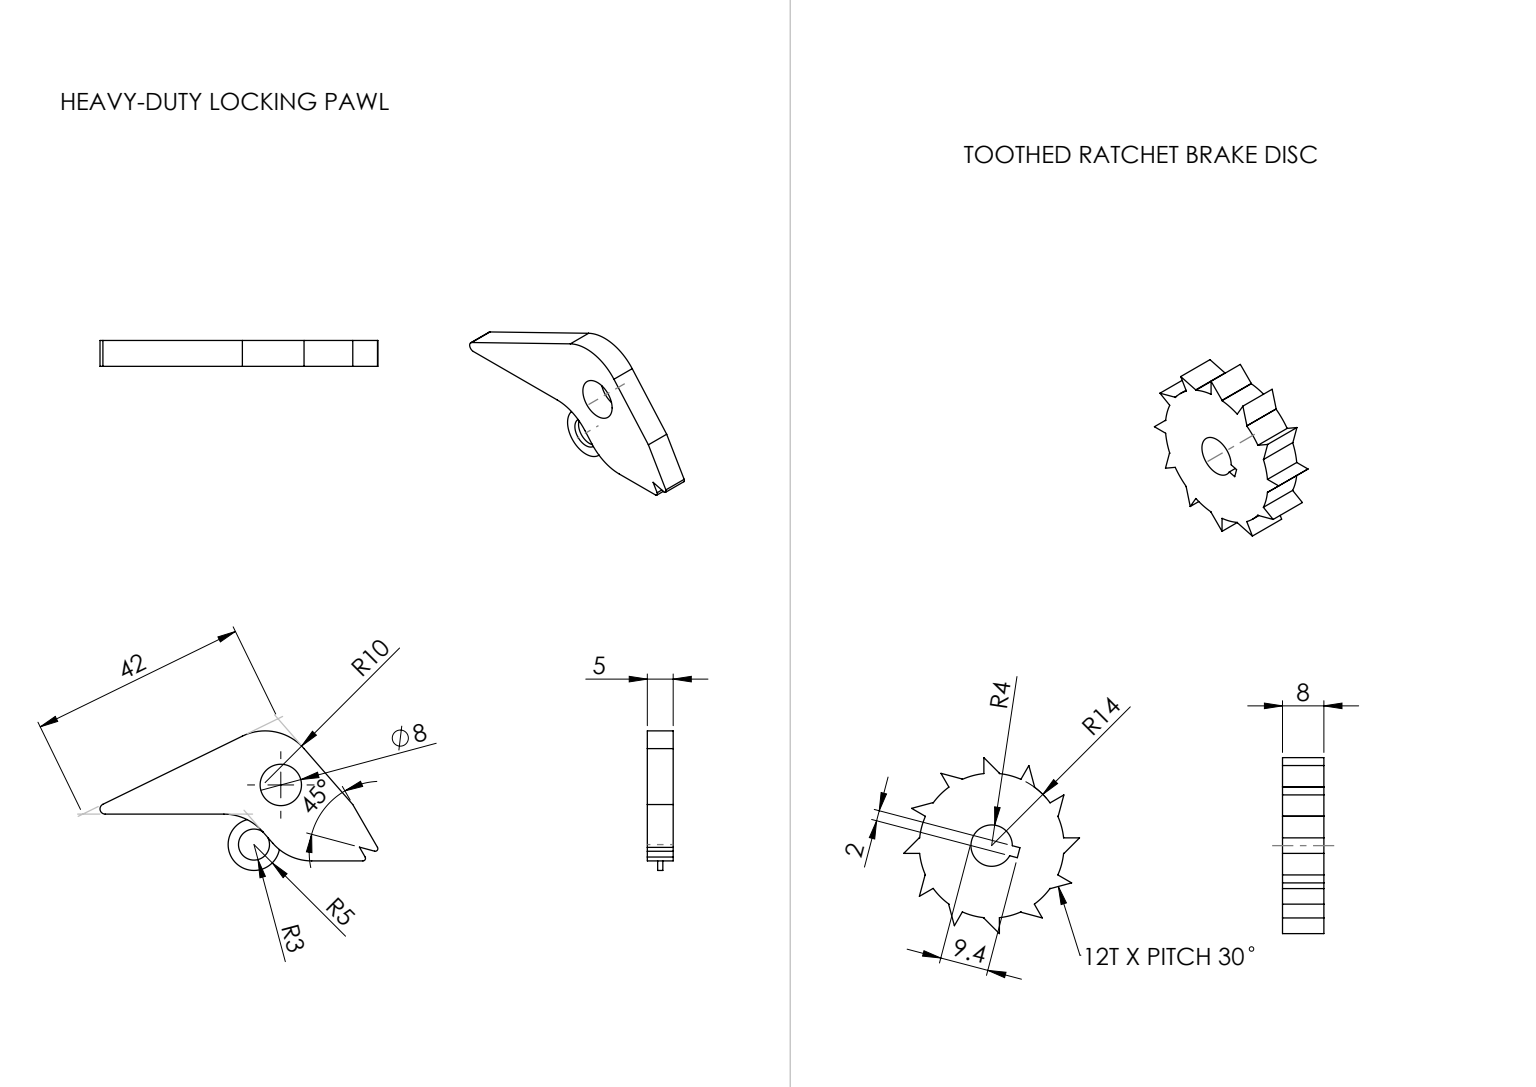
ISO-10303-21;
HEADER;
FILE_DESCRIPTION (('STEP AP214'),
    '1' );
FILE_NAME ('Heavy-Duty Locking Pawl.step',
    '2026-09-28T15:49:00',
    ( '' ),
    ( '' ),
    'SwSTEP 2.0',
    'SolidWorks 2026',
    '' );
FILE_SCHEMA (( 'AUTOMOTIVE_DESIGN' ));
ENDSEC;

DATA;
#126=LINE ( 'NONE', #14327, #30319 ) ;
#160=CARTESIAN_POINT ( 'NONE',  ( -39.49999999999999289, -4.676198662292047281, 104.0227405789415798 ) ) ;
#179=ORIENTED_EDGE ( 'NONE', *, *, #27489, .F. ) ;
#216=DIRECTION ( 'NONE',  ( 0.000000000000000000, -0.4387576694191721027, 0.8986054237126862576 ) ) ;
#291=DIRECTION ( 'NONE',  ( 1.000000000000000000, 0.000000000000000000, 0.000000000000000000 ) ) ;
#309=PLANE ( 'NONE',  #1960 ) ;
#345=ADVANCED_FACE ( 'NONE', ( #24395 ), #13584, .T. ) ;
#411=VECTOR ( 'NONE', #24803, 1000.000000000000000 ) ;
#434=ADVANCED_FACE ( 'NONE', ( #13768 ), #33029, .T. ) ;
#439=AXIS2_PLACEMENT_3D ( 'NONE', #27809, #6356, #14099 ) ;
#451=SURFACE_SIDE_STYLE ('',( #22398 ) ) ;
#476=DIRECTION ( 'NONE',  ( 0.000000000000000000, -1.000000000000000000, -2.543449303551180694E-16 ) ) ;
#492=ADVANCED_FACE ( 'NONE', ( #19665 ), #33908, .F. ) ;
#518=CARTESIAN_POINT ( 'NONE',  ( -37.49999999999999289, -11.52052244843579309, 112.1848168619253840 ) ) ;
#555=CARTESIAN_POINT ( 'NONE',  ( -39.49999999999999289, -3.784235812937200460, 96.08311962715481513 ) ) ;
#666=EDGE_CURVE ( 'NONE', #20493, #13129, #4578, .T. ) ;
#702=EDGE_CURVE ( 'NONE', #28348, #19239, #12841, .T. ) ;
#733=ORIENTED_EDGE ( 'NONE', *, *, #666, .T. ) ;
#827=EDGE_CURVE ( 'NONE', #17814, #16992, #7429, .T. ) ;
#850=CARTESIAN_POINT ( 'NONE',  ( -36.49999999999999289, -11.52052244843579309, 115.1848168619253698 ) ) ;
#935=CIRCLE ( 'NONE', #21042, 4.000000000000003553 ) ;
#968=CARTESIAN_POINT ( 'NONE',  ( -39.49999999999999289, -12.06102132296306451, 91.30451528491657598 ) ) ;
#983=DIRECTION ( 'NONE',  ( 0.000000000000000000, 0.000000000000000000, -1.000000000000000000 ) ) ;
#995=CIRCLE ( 'NONE', #24010, 2.999999999999988898 ) ;
#1085=ORIENTED_EDGE ( 'NONE', *, *, #11721, .T. ) ;
#1092=CARTESIAN_POINT ( 'NONE',  ( -39.49999999999999289, -13.92619866229204106, 93.69175626110634880 ) ) ;
#1100=DIRECTION ( 'NONE',  ( 1.000000000000000000, 0.000000000000000000, 0.000000000000000000 ) ) ;
#1146=DIRECTION ( 'NONE',  ( -1.000000000000000000, -0.000000000000000000, -0.000000000000000000 ) ) ;
#1153=AXIS2_PLACEMENT_3D ( 'NONE', #33101, #33441, #33277 ) ;
#1171=DIRECTION ( 'NONE',  ( 0.000000000000000000, 0.000000000000000000, -1.000000000000000000 ) ) ;
#1328=ADVANCED_FACE ( 'NONE', ( #12443 ), #23786, .F. ) ;
#1343=DIRECTION ( 'NONE',  ( -0.000000000000000000, 1.611597878369477150E-16, -1.000000000000000000 ) ) ;
#1392=ORIENTED_EDGE ( 'NONE', *, *, #8153, .T. ) ;
#1416=EDGE_LOOP ( 'NONE', ( #5626, #28974, #6098, #6104 ) ) ;
#1434=DIRECTION ( 'NONE',  ( 0.000000000000000000, 0.000000000000000000, -1.000000000000000000 ) ) ;
#1472=ORIENTED_EDGE ( 'NONE', *, *, #16597, .F. ) ;
#1475=DIRECTION ( 'NONE',  ( 0.000000000000000000, 0.000000000000000000, 1.000000000000000000 ) ) ;
#1494=CARTESIAN_POINT ( 'NONE',  ( -34.49999999999998579, 0.4463568765849662556, 113.0433323525902125 ) ) ;
#1529=VECTOR ( 'NONE', #28337, 1000.000000000000000 ) ;
#1682=CARTESIAN_POINT ( 'NONE',  ( -36.99999999999999289, -6.699660887819688604, 116.5112005972652014 ) ) ;
#1749=EDGE_LOOP ( 'NONE', ( #26063, #16857, #20128, #5547 ) ) ;
#1756=CARTESIAN_POINT ( 'NONE',  ( -34.49999999999998579, -5.633167542791597704, 143.9590043477703887 ) ) ;
#1773=MECHANICAL_DESIGN_GEOMETRIC_PRESENTATION_REPRESENTATION('',(#5255),#9237);
#1785=VERTEX_POINT ( 'NONE', #20655 ) ;
#1808=LINE ( 'NONE', #20507, #17106 ) ;
#1900=AXIS2_PLACEMENT_3D ( 'NONE', #29623, #32852, #8343 ) ;
#1924=VERTEX_POINT ( 'NONE', #21543 ) ;
#1934=VERTEX_POINT ( 'NONE', #24451 ) ;
#1948=FACE_OUTER_BOUND ( 'NONE', #6910, .T. ) ;
#1960=AXIS2_PLACEMENT_3D ( 'NONE', #2687, #5893, #33431 ) ;
#2069=ORIENTED_EDGE ( 'NONE', *, *, #2492, .T. ) ;
#2127=FACE_OUTER_BOUND ( 'NONE', #12727, .T. ) ;
#2140=CARTESIAN_POINT ( 'NONE',  ( -39.49999999999999289, -13.10640646055107084, 90.70096189432331357 ) ) ;
#2179=FACE_OUTER_BOUND ( 'NONE', #13270, .T. ) ;
#2257=VECTOR ( 'NONE', #1343, 1000.000000000000000 ) ;
#2271=CARTESIAN_POINT ( 'NONE',  ( -36.49999999999999289, -12.47865190846804495, 110.2774766518096925 ) ) ;
#2395=CYLINDRICAL_SURFACE ( 'NONE', #17961, 0.5000000000000004441 ) ;
#2423=ORIENTED_EDGE ( 'NONE', *, *, #24195, .T. ) ;
#2471=ORIENTED_EDGE ( 'NONE', *, *, #34763, .F. ) ;
#2474=DIRECTION ( 'NONE',  ( 0.000000000000000000, 0.000000000000000000, -1.000000000000000000 ) ) ;
#2492=EDGE_CURVE ( 'NONE', #8765, #31548, #12899, .T. ) ;
#2501=SURFACE_SIDE_STYLE ('',( #10769 ) ) ;
#2507=EDGE_CURVE ( 'NONE', #26405, #1934, #8015, .T. ) ;
#2585=ORIENTED_EDGE ( 'NONE', *, *, #25973, .T. ) ;
#2670=EDGE_LOOP ( 'NONE', ( #20970, #14422, #16376, #5466, #10981, #179, #16771, #20477, #24151, #2069 ) ) ;
#2678=LINE ( 'NONE', #13302, #14269 ) ;
#2687=CARTESIAN_POINT ( 'NONE',  ( -39.49999999999999289, -14.67619866229204284, 93.25874355921412473 ) ) ;
#2691=CIRCLE ( 'NONE', #10149, 0.5000000000000004441 ) ;
#2799=COLOUR_RGB ( '', 0.09019608, 0.27058824, 0.51372549) ;
#2846=CARTESIAN_POINT ( 'NONE',  ( -37.49999999999999289, -4.676198662292047281, 104.0227405789415798 ) ) ;
#2848=FACE_OUTER_BOUND ( 'NONE', #11113, .T. ) ;
#2882=ADVANCED_FACE ( 'NONE', ( #34281 ), #28876, .F. ) ;
#2893=AXIS2_PLACEMENT_3D ( 'NONE', #19566, #5902, #6080 ) ;
#2973=CARTESIAN_POINT ( 'NONE',  ( -36.49999999999999289, -11.52052244843579309, 115.1848168619253698 ) ) ;
#3057=LINE ( 'NONE', #518, #22680 ) ;
#3058=AXIS2_PLACEMENT_3D ( 'NONE', #21859, #4960, #29980 ) ;
#3076=CARTESIAN_POINT ( 'NONE',  ( -37.49999999999999289, -11.52052244843579309, 115.1848168619253698 ) ) ;
#3128=LINE ( 'NONE', #14606, #28088 ) ;
#3134=CARTESIAN_POINT ( 'NONE',  ( -39.49999999999999289, -9.059673409587547965, 113.4689433211305811 ) ) ;
#3166=( LENGTH_UNIT ( ) NAMED_UNIT ( * ) SI_UNIT ( .MILLI., .METRE. ) );
#3186=CIRCLE ( 'NONE', #10057, 0.5000000000000004441 ) ;
#3275=LINE ( 'NONE', #555, #6619 ) ;
#3290=LINE ( 'NONE', #22523, #14750 ) ;
#3350=( NAMED_UNIT ( * ) SI_UNIT ( $, .STERADIAN. ) SOLID_ANGLE_UNIT ( ) );
#3355=ADVANCED_FACE ( 'NONE', ( #16034 ), #2395, .T. ) ;
#3380=( GEOMETRIC_REPRESENTATION_CONTEXT ( 3 ) GLOBAL_UNCERTAINTY_ASSIGNED_CONTEXT ( ( #13929 ) ) GLOBAL_UNIT_ASSIGNED_CONTEXT ( ( #15783, #35436, #7692 ) ) REPRESENTATION_CONTEXT ( 'NONE', 'WORKASPACE' ) );
#3399=CIRCLE ( 'NONE', #17732, 0.5000000000000004441 ) ;
#3415=FACE_OUTER_BOUND ( 'NONE', #21315, .T. ) ;
#3486=CARTESIAN_POINT ( 'NONE',  ( -34.49999999999998579, -1.338792908815551458E-14, 114.0000000000000000 ) ) ;
#3550=EDGE_CURVE ( 'NONE', #1924, #18506, #17453, .T. ) ;
#3609=EDGE_LOOP ( 'NONE', ( #6893, #13089, #3660, #8012 ) ) ;
#3660=ORIENTED_EDGE ( 'NONE', *, *, #8778, .T. ) ;
#3760=ORIENTED_EDGE ( 'NONE', *, *, #24701, .T. ) ;
#3767=ORIENTED_EDGE ( 'NONE', *, *, #3550, .T. ) ;
#3815=ORIENTED_EDGE ( 'NONE', *, *, #827, .F. ) ;
#3950=ADVANCED_BREP_SHAPE_REPRESENTATION ( '', ( #33931, #21307 ), #6954 ) ;
#4036=EDGE_CURVE ( 'NONE', #4537, #12439, #11122, .T. ) ;
#4087=CARTESIAN_POINT ( 'NONE',  ( -39.49999999999999289, -9.059673409587547965, 113.4689433211305811 ) ) ;
#4113=CARTESIAN_POINT ( 'NONE',  ( -34.49999999999998579, -13.10640646055107084, 90.70096189432331357 ) ) ;
#4135=ORIENTED_EDGE ( 'NONE', *, *, #2507, .T. ) ;
#4175=LINE ( 'NONE', #15115, #16469 ) ;
#4216=DIRECTION ( 'NONE',  ( 1.000000000000000000, 0.000000000000000000, 0.000000000000000000 ) ) ;
#4221=CYLINDRICAL_SURFACE ( 'NONE', #5807, 2.999999999999988898 ) ;
#4229=DIRECTION ( 'NONE',  ( 1.000000000000000000, 0.000000000000000000, 0.000000000000000000 ) ) ;
#4263=CYLINDRICAL_SURFACE ( 'NONE', #33096, 9.999999999999994671 ) ;
#4332=DIRECTION ( 'NONE',  ( 1.000000000000000000, 0.000000000000000000, 0.000000000000000000 ) ) ;
#4342=DIRECTION ( 'NONE',  ( 0.000000000000000000, 0.000000000000000000, -1.000000000000000000 ) ) ;
#4358=CARTESIAN_POINT ( 'NONE',  ( -34.49999999999998579, -14.67619866229204284, 93.25874355921412473 ) ) ;
#4434=AXIS2_PLACEMENT_3D ( 'NONE', #13073, #9996, #26752 ) ;
#4438=EDGE_CURVE ( 'NONE', #4619, #31088, #17539, .T. ) ;
#4454=EDGE_CURVE ( 'NONE', #5280, #20493, #26103, .T. ) ;
#4487=VECTOR ( 'NONE', #23615, 1000.000000000000227 ) ;
#4510=CARTESIAN_POINT ( 'NONE',  ( -37.49999999999999289, -9.059673409587521320, 113.4689433211306095 ) ) ;
#4524=PLANE ( 'NONE',  #35139 ) ;
#4537=VERTEX_POINT ( 'NONE', #2271 ) ;
#4578=LINE ( 'NONE', #1682, #13404 ) ;
#4582=FACE_OUTER_BOUND ( 'NONE', #13992, .T. ) ;
#4600=LINE ( 'NONE', #20394, #2257 ) ;
#4619=VERTEX_POINT ( 'NONE', #7103 ) ;
#4626=DIRECTION ( 'NONE',  ( 0.000000000000000000, 0.000000000000000000, -1.000000000000000000 ) ) ;
#4844=ORIENTED_EDGE ( 'NONE', *, *, #15258, .T. ) ;
#4888=ADVANCED_FACE ( 'NONE', ( #28460 ), #28993, .F. ) ;
#4960=DIRECTION ( 'NONE',  ( 1.000000000000000000, 0.000000000000000000, 0.000000000000000000 ) ) ;
#5006=DIRECTION ( 'NONE',  ( 1.000000000000000000, 0.000000000000000000, 0.000000000000000000 ) ) ;
#5017=ORIENTED_EDGE ( 'NONE', *, *, #2507, .F. ) ;
#5086=ORIENTED_EDGE ( 'NONE', *, *, #7009, .T. ) ;
#5134=CARTESIAN_POINT ( 'NONE',  ( -39.49999999999999289, -12.06102132296306451, 91.30451528491657598 ) ) ;
#5159=CARTESIAN_POINT ( 'NONE',  ( -34.49999999999998579, -12.31102132296306451, 91.23752798680880005 ) ) ;
#5177=CARTESIAN_POINT ( 'NONE',  ( -39.49999999999999289, 0.4463568765849662556, 113.0433323525902125 ) ) ;
#5192=CARTESIAN_POINT ( 'NONE',  ( -37.49999999999999289, -11.52052244843579309, 118.1848168619253556 ) ) ;
#5249=EDGE_CURVE ( 'NONE', #13216, #19089, #3057, .T. ) ;
#5255=STYLED_ITEM ( 'NONE', ( #25657 ), #3950 ) ;
#5280=VERTEX_POINT ( 'NONE', #11665 ) ;
#5287=VERTEX_POINT ( 'NONE', #8960 ) ;
#5289=EDGE_CURVE ( 'NONE', #12439, #23662, #25197, .T. ) ;
#5301=ADVANCED_FACE ( 'NONE', ( #3415 ), #14363, .T. ) ;
#5365=PLANE ( 'NONE',  #12648 ) ;
#5427=CARTESIAN_POINT ( 'NONE',  ( -34.49999999999998579, -12.06102132296306451, 91.30451528491657598 ) ) ;
#5435=CARTESIAN_POINT ( 'NONE',  ( -39.49999999999999289, -13.92619866229204106, 93.69175626110634880 ) ) ;
#5466=ORIENTED_EDGE ( 'NONE', *, *, #5289, .F. ) ;
#5501=AXIS2_PLACEMENT_3D ( 'NONE', #15560, #20609, #31609 ) ;
#5547=ORIENTED_EDGE ( 'NONE', *, *, #15003, .F. ) ;
#5568=AXIS2_PLACEMENT_3D ( 'NONE', #7028, #18002, #28999 ) ;
#5587=EDGE_CURVE ( 'NONE', #12439, #29235, #29850, .T. ) ;
#5620=DIRECTION ( 'NONE',  ( 1.000000000000000000, 0.000000000000000000, 0.000000000000000000 ) ) ;
#5626=ORIENTED_EDGE ( 'NONE', *, *, #702, .F. ) ;
#5687=ORIENTED_EDGE ( 'NONE', *, *, #32711, .T. ) ;
#5715=EDGE_LOOP ( 'NONE', ( #13468, #17776, #8108, #12400 ) ) ;
#5734=EDGE_CURVE ( 'NONE', #5280, #19239, #9485, .T. ) ;
#5771=ORIENTED_EDGE ( 'NONE', *, *, #10603, .T. ) ;
#5772=EDGE_CURVE ( 'NONE', #32244, #10765, #19268, .T. ) ;
#5773=LINE ( 'NONE', #8280, #6186 ) ;
#5807=AXIS2_PLACEMENT_3D ( 'NONE', #14992, #23827, #32105 ) ;
#5819=ORIENTED_EDGE ( 'NONE', *, *, #17002, .F. ) ;
#5827=AXIS2_PLACEMENT_3D ( 'NONE', #22811, #9319, #30749 ) ;
#5837=CARTESIAN_POINT ( 'NONE',  ( -39.49999999999999289, -1.387778780781445676E-14, 110.0000000000000000 ) ) ;
#5876=ADVANCED_FACE ( 'NONE', ( #31251 ), #14858, .F. ) ;
#5882=PLANE ( 'NONE',  #28566 ) ;
#5893=DIRECTION ( 'NONE',  ( 0.000000000000000000, 0.5000000000000012212, -0.8660254037844380415 ) ) ;
#5902=DIRECTION ( 'NONE',  ( 0.000000000000000000, -1.000000000000000000, -1.611597878369477150E-16 ) ) ;
#5952=EDGE_CURVE ( 'NONE', #14078, #1924, #10657, .T. ) ;
#5988=AXIS2_PLACEMENT_3D ( 'NONE', #17689, #25986, #20191 ) ;
#6029=ORIENTED_EDGE ( 'NONE', *, *, #16523, .T. ) ;
#6044=CLOSED_SHELL ( 'NONE', ( #31093, #345, #11165, #5876, #2882, #5301, #31535, #1328, #13097, #434, #30007, #33069, #10334, #20487, #27405, #19750, #19706, #9581, #492, #35008, #17406, #7272, #29548, #4888, #24247, #3355 ) ) ;
#6050=VECTOR ( 'NONE', #30202, 1000.000000000000000 ) ;
#6080=DIRECTION ( 'NONE',  ( 0.000000000000000000, 1.611597878369477150E-16, -1.000000000000000000 ) ) ;
#6098=ORIENTED_EDGE ( 'NONE', *, *, #15711, .T. ) ;
#6104=ORIENTED_EDGE ( 'NONE', *, *, #5734, .T. ) ;
#6115=DIRECTION ( 'NONE',  ( 0.000000000000000000, 0.000000000000000000, -1.000000000000000000 ) ) ;
#6128=VECTOR ( 'NONE', #33076, 1000.000000000000114 ) ;
#6150=CARTESIAN_POINT ( 'NONE',  ( -37.49999999999999289, -9.059673409587547965, 113.4689433211305811 ) ) ;
#6186=VECTOR ( 'NONE', #19769, 1000.000000000000000 ) ;
#6272=ORIENTED_EDGE ( 'NONE', *, *, #28436, .T. ) ;
#6275=AXIS2_PLACEMENT_3D ( 'NONE', #18654, #24609, #35596 ) ;
#6329=DIRECTION ( 'NONE',  ( -0.000000000000000000, 1.611597878369477150E-16, -1.000000000000000000 ) ) ;
#6355=VECTOR ( 'NONE', #20571, 1000.000000000000000 ) ;
#6356=DIRECTION ( 'NONE',  ( 1.000000000000000000, 0.000000000000000000, 0.000000000000000000 ) ) ;
#6366=EDGE_CURVE ( 'NONE', #11436, #13129, #18144, .T. ) ;
#6393=LINE ( 'NONE', #33769, #7622 ) ;
#6394=DIRECTION ( 'NONE',  ( 0.000000000000000000, 0.000000000000000000, -1.000000000000000000 ) ) ;
#6599=AXIS2_PLACEMENT_3D ( 'NONE', #2846, #10935, #8218 ) ;
#6619=VECTOR ( 'NONE', #22508, 1000.000000000000000 ) ;
#6668=ORIENTED_EDGE ( 'NONE', *, *, #7227, .T. ) ;
#6700=AXIS2_PLACEMENT_3D ( 'NONE', #29243, #21109, #29416 ) ;
#6708=FACE_OUTER_BOUND ( 'NONE', #7538, .T. ) ;
#6782=SHAPE_DEFINITION_REPRESENTATION ( #23303, #33958 ) ;
#6805=ORIENTED_EDGE ( 'NONE', *, *, #20272, .T. ) ;
#6837=DIRECTION ( 'NONE',  ( -1.000000000000000000, -0.000000000000000000, -0.000000000000000000 ) ) ;
#6875=CARTESIAN_POINT ( 'NONE',  ( -34.49999999999998579, -4.676198662292047281, 104.0227405789415798 ) ) ;
#6880=CIRCLE ( 'NONE', #27024, 2.999999999999988898 ) ;
#6893=ORIENTED_EDGE ( 'NONE', *, *, #22907, .F. ) ;
#6905=CARTESIAN_POINT ( 'NONE',  ( -39.49999999999999289, -12.79398423610758684, 91.86693750936007064 ) ) ;
#6910=EDGE_LOOP ( 'NONE', ( #24221, #6805, #4135, #5086 ) ) ;
#6911=ORIENTED_EDGE ( 'NONE', *, *, #29058, .T. ) ;
#6914=VERTEX_POINT ( 'NONE', #20334 ) ;
#6930=DIRECTION ( 'NONE',  ( 1.000000000000000000, 0.000000000000000000, 0.000000000000000000 ) ) ;
#6954=( GEOMETRIC_REPRESENTATION_CONTEXT ( 3 ) GLOBAL_UNCERTAINTY_ASSIGNED_CONTEXT ( ( #28323 ) ) GLOBAL_UNIT_ASSIGNED_CONTEXT ( ( #3166, #22227, #24947 ) ) REPRESENTATION_CONTEXT ( 'NONE', 'WORKASPACE' ) );
#6960=ORIENTED_EDGE ( 'NONE', *, *, #7245, .F. ) ;
#7009=EDGE_CURVE ( 'NONE', #1934, #13123, #31166, .T. ) ;
#7028=CARTESIAN_POINT ( 'NONE',  ( -36.49999999999999289, -11.52052244843579309, 115.1848168619253698 ) ) ;
#7086=AXIS2_PLACEMENT_3D ( 'NONE', #31849, #12598, #9881 ) ;
#7103=CARTESIAN_POINT ( 'NONE',  ( -39.49999999999999289, -1.387778780781445676E-14, 106.0000000000000000 ) ) ;
#7227=EDGE_CURVE ( 'NONE', #7877, #20597, #4175, .T. ) ;
#7245=EDGE_CURVE ( 'NONE', #19089, #23662, #17027, .T. ) ;
#7272=ADVANCED_FACE ( 'NONE', ( #11288 ), #5882, .T. ) ;
#7289=AXIS2_PLACEMENT_3D ( 'NONE', #19639, #19808, #30481 ) ;
#7341=EDGE_CURVE ( 'NONE', #14392, #14078, #25156, .T. ) ;
#7362=EDGE_CURVE ( 'NONE', #11298, #33791, #126, .T. ) ;
#7376=MECHANICAL_DESIGN_GEOMETRIC_PRESENTATION_REPRESENTATION('',(#22884),#3380);
#7426=ORIENTED_EDGE ( 'NONE', *, *, #20550, .F. ) ;
#7429=LINE ( 'NONE', #17868, #21456 ) ;
#7433=CARTESIAN_POINT ( 'NONE',  ( -34.49999999999998579, -13.10640646055107084, 90.70096189432331357 ) ) ;
#7520=DIRECTION ( 'NONE',  ( 1.000000000000000000, 0.000000000000000000, 0.000000000000000000 ) ) ;
#7533=DIRECTION ( 'NONE',  ( 1.000000000000000000, 0.000000000000000000, 0.000000000000000000 ) ) ;
#7538=EDGE_LOOP ( 'NONE', ( #13140, #18016, #8020, #16187 ) ) ;
#7616=ORIENTED_EDGE ( 'NONE', *, *, #8153, .F. ) ;
#7622=VECTOR ( 'NONE', #17357, 1000.000000000000000 ) ;
#7644=FACE_OUTER_BOUND ( 'NONE', #3609, .T. ) ;
#7692=( NAMED_UNIT ( * ) SI_UNIT ( $, .STERADIAN. ) SOLID_ANGLE_UNIT ( ) );
#7762=AXIS2_PLACEMENT_3D ( 'NONE', #34316, #9109, #23315 ) ;
#7824=DIRECTION ( 'NONE',  ( 1.000000000000000000, 0.000000000000000000, 0.000000000000000000 ) ) ;
#7834=CARTESIAN_POINT ( 'NONE',  ( -39.49999999999999289, -11.24969279549607748, 111.5585998451919778 ) ) ;
#7866=ORIENTED_EDGE ( 'NONE', *, *, #33945, .T. ) ;
#7874=VECTOR ( 'NONE', #216, 1000.000000000000227 ) ;
#7877=VERTEX_POINT ( 'NONE', #1756 ) ;
#7915=ORIENTED_EDGE ( 'NONE', *, *, #28625, .T. ) ;
#7927=AXIS2_PLACEMENT_3D ( 'NONE', #3076, #27903, #14031 ) ;
#8012=ORIENTED_EDGE ( 'NONE', *, *, #7362, .T. ) ;
#8015=LINE ( 'NONE', #20969, #34667 ) ;
#8020=ORIENTED_EDGE ( 'NONE', *, *, #20272, .F. ) ;
#8043=CARTESIAN_POINT ( 'NONE',  ( -34.49999999999998579, -12.31102132296306451, 91.73752798680880005 ) ) ;
#8078=VECTOR ( 'NONE', #34498, 1000.000000000000114 ) ;
#8108=ORIENTED_EDGE ( 'NONE', *, *, #3550, .F. ) ;
#8153=EDGE_CURVE ( 'NONE', #4619, #17814, #10219, .T. ) ;
#8217=DIRECTION ( 'NONE',  ( 0.000000000000000000, 0.000000000000000000, -1.000000000000000000 ) ) ;
#8218=DIRECTION ( 'NONE',  ( 0.000000000000000000, -6.245004513516508695E-15, -1.000000000000000000 ) ) ;
#8280=CARTESIAN_POINT ( 'NONE',  ( -34.49999999999998579, -3.784235812937200460, 96.08311962715481513 ) ) ;
#8343=DIRECTION ( 'NONE',  ( 0.000000000000000000, -0.2588190451025194072, -0.9659258262890686453 ) ) ;
#8355=CIRCLE ( 'NONE', #22156, 2.999999999999988898 ) ;
#8528=FACE_OUTER_BOUND ( 'NONE', #27433, .T. ) ;
#8532=CARTESIAN_POINT ( 'NONE',  ( -39.49999999999999289, -12.00833024919777081, 94.79903810567661537 ) ) ;
#8588=CARTESIAN_POINT ( 'NONE',  ( -39.49999999999999289, -11.24969279549607748, 111.5585998451919778 ) ) ;
#8595=FACE_OUTER_BOUND ( 'NONE', #21731, .T. ) ;
#8683=CIRCLE ( 'NONE', #18454, 9.999999999999994671 ) ;
#8696=DIRECTION ( 'NONE',  ( 0.000000000000000000, 0.000000000000000000, -1.000000000000000000 ) ) ;
#8713=ORIENTED_EDGE ( 'NONE', *, *, #14812, .F. ) ;
#8765=VERTEX_POINT ( 'NONE', #31115 ) ;
#8778=EDGE_CURVE ( 'NONE', #6914, #11298, #10753, .T. ) ;
#8886=DIRECTION ( 'NONE',  ( 1.000000000000000000, 0.000000000000000000, 0.000000000000000000 ) ) ;
#8897=( NAMED_UNIT ( * ) PLANE_ANGLE_UNIT ( ) SI_UNIT ( $, .RADIAN. ) );
#8957=DIRECTION ( 'NONE',  ( 0.000000000000000000, 0.000000000000000000, -1.000000000000000000 ) ) ;
#8960=CARTESIAN_POINT ( 'NONE',  ( -34.49999999999998579, -9.059673409587547965, 113.4689433211305811 ) ) ;
#8991=ORIENTED_EDGE ( 'NONE', *, *, #4036, .T. ) ;
#9033=ORIENTED_EDGE ( 'NONE', *, *, #33049, .T. ) ;
#9109=DIRECTION ( 'NONE',  ( 1.000000000000000000, 0.000000000000000000, 0.000000000000000000 ) ) ;
#9154=ORIENTED_EDGE ( 'NONE', *, *, #9253, .T. ) ;
#9212=CARTESIAN_POINT ( 'NONE',  ( -39.49999999999999289, -13.10640646055107084, 90.70096189432331357 ) ) ;
#9237=( GEOMETRIC_REPRESENTATION_CONTEXT ( 3 ) GLOBAL_UNCERTAINTY_ASSIGNED_CONTEXT ( ( #31195 ) ) GLOBAL_UNIT_ASSIGNED_CONTEXT ( ( #14468, #8897, #3350 ) ) REPRESENTATION_CONTEXT ( 'NONE', 'WORKASPACE' ) );
#9253=EDGE_CURVE ( 'NONE', #7877, #12138, #10751, .T. ) ;
#9265=EDGE_CURVE ( 'NONE', #26405, #26937, #13659, .T. ) ;
#9268=CARTESIAN_POINT ( 'NONE',  ( -39.49999999999999289, -12.31102132296306451, 91.73752798680880005 ) ) ;
#9319=DIRECTION ( 'NONE',  ( -1.000000000000000000, -0.000000000000000000, -0.000000000000000000 ) ) ;
#9375=CIRCLE ( 'NONE', #7086, 0.5000000000000004441 ) ;
#9402=DIRECTION ( 'NONE',  ( -0.000000000000000000, 0.8986054237126863686, 0.4387576694191721027 ) ) ;
#9456=DIRECTION ( 'NONE',  ( 0.000000000000000000, 0.000000000000000000, -1.000000000000000000 ) ) ;
#9485=CIRCLE ( 'NONE', #23895, 2.999999999999988898 ) ;
#9488=DIRECTION ( 'NONE',  ( 0.000000000000000000, 0.8660254037844381525, 0.5000000000000006661 ) ) ;
#9508=ORIENTED_EDGE ( 'NONE', *, *, #27164, .F. ) ;
#9581=ADVANCED_FACE ( 'NONE', ( #33724, #8528 ), #33373, .T. ) ;
#9585=CIRCLE ( 'NONE', #28550, 4.000000000000003553 ) ;
#9651=CARTESIAN_POINT ( 'NONE',  ( -37.49999999999999289, -11.52052244843579309, 115.1848168619253698 ) ) ;
#9663=DIRECTION ( 'NONE',  ( -0.000000000000000000, 0.7535859266250379829, 0.6573494133204068612 ) ) ;
#9677=DIRECTION ( 'NONE',  ( 0.000000000000000000, 0.000000000000000000, -1.000000000000000000 ) ) ;
#9701=CIRCLE ( 'NONE', #25834, 9.999999999999994671 ) ;
#9735=DIRECTION ( 'NONE',  ( -0.000000000000000000, 2.543449303551180694E-16, -1.000000000000000000 ) ) ;
#9770=CYLINDRICAL_SURFACE ( 'NONE', #5988, 0.5000000000000004441 ) ;
#9881=DIRECTION ( 'NONE',  ( 0.000000000000000000, 0.000000000000000000, -1.000000000000000000 ) ) ;
#9947=ORIENTED_EDGE ( 'NONE', *, *, #15003, .T. ) ;
#9994=CIRCLE ( 'NONE', #34732, 4.999999999999990230 ) ;
#9996=DIRECTION ( 'NONE',  ( -1.000000000000000000, -0.000000000000000000, -0.000000000000000000 ) ) ;
#10002=DIRECTION ( 'NONE',  ( 1.000000000000000000, 0.000000000000000000, 0.000000000000000000 ) ) ;
#10057=AXIS2_PLACEMENT_3D ( 'NONE', #32193, #7520, #18499 ) ;
#10149=AXIS2_PLACEMENT_3D ( 'NONE', #8043, #291, #8217 ) ;
#10179=ORIENTED_EDGE ( 'NONE', *, *, #5772, .T. ) ;
#10219=CIRCLE ( 'NONE', #29199, 4.000000000000003553 ) ;
#10334=ADVANCED_FACE ( 'NONE', ( #2848 ), #5365, .T. ) ;
#10495=CARTESIAN_POINT ( 'NONE',  ( -39.49999999999999289, 9.432411113711806294, 117.4309090467819772 ) ) ;
#10505=VECTOR ( 'NONE', #16102, 1000.000000000000000 ) ;
#10524=EDGE_LOOP ( 'NONE', ( #18600, #28082, #28258, #30946 ) ) ;
#10589=FILL_AREA_STYLE_COLOUR ( '', #2799 ) ;
#10596=LINE ( 'NONE', #4510, #32095 ) ;
#10603=EDGE_CURVE ( 'NONE', #18506, #26302, #24226, .T. ) ;
#10657=CIRCLE ( 'NONE', #15224, 0.5000000000000004441 ) ;
#10681=CARTESIAN_POINT ( 'NONE',  ( -39.49999999999999289, -1.387778780781445676E-14, 110.0000000000000000 ) ) ;
#10741=CARTESIAN_POINT ( 'NONE',  ( -36.49999999999999289, -11.24969279549607748, 111.5585998451919778 ) ) ;
#10751=LINE ( 'NONE', #13285, #30894 ) ;
#10753=CIRCLE ( 'NONE', #17049, 9.999999999999994671 ) ;
#10765=VERTEX_POINT ( 'NONE', #19333 ) ;
#10769=SURFACE_STYLE_FILL_AREA ( #30038 ) ;
#10865=DIRECTION ( 'NONE',  ( 1.000000000000000000, 0.000000000000000000, 0.000000000000000000 ) ) ;
#10877=CARTESIAN_POINT ( 'NONE',  ( -34.49999999999998579, -12.79398423610758684, 91.86693750936007064 ) ) ;
#10922=FACE_BOUND ( 'NONE', #17086, .T. ) ;
#10935=DIRECTION ( 'NONE',  ( -1.000000000000000000, -0.000000000000000000, -0.000000000000000000 ) ) ;
#10981=ORIENTED_EDGE ( 'NONE', *, *, #5587, .T. ) ;
#11074=CARTESIAN_POINT ( 'NONE',  ( -37.49999999999999289, -11.52052244843579309, 115.1848168619253698 ) ) ;
#11092=EDGE_CURVE ( 'NONE', #26408, #16117, #32283, .T. ) ;
#11113=EDGE_LOOP ( 'NONE', ( #23557, #9154, #7866, #25493 ) ) ;
#11122=CIRCLE ( 'NONE', #19180, 9.999999999999994671 ) ;
#11131=DIRECTION ( 'NONE',  ( 0.000000000000000000, -0.6573494133204068612, 0.7535859266250379829 ) ) ;
#11165=ADVANCED_FACE ( 'NONE', ( #4582 ), #4221, .F. ) ;
#11288=FACE_OUTER_BOUND ( 'NONE', #22352, .T. ) ;
#11298=VERTEX_POINT ( 'NONE', #10495 ) ;
#11380=ORIENTED_EDGE ( 'NONE', *, *, #22907, .T. ) ;
#11397=ORIENTED_EDGE ( 'NONE', *, *, #33945, .F. ) ;
#11436=VERTEX_POINT ( 'NONE', #6150 ) ;
#11498=DIRECTION ( 'NONE',  ( 1.000000000000000000, 0.000000000000000000, 0.000000000000000000 ) ) ;
#11518=VECTOR ( 'NONE', #16072, 1000.000000000000000 ) ;
#11559=FACE_OUTER_BOUND ( 'NONE', #1749, .T. ) ;
#11572=ORIENTED_EDGE ( 'NONE', *, *, #11092, .T. ) ;
#11634=ORIENTED_EDGE ( 'NONE', *, *, #27086, .T. ) ;
#11665=CARTESIAN_POINT ( 'NONE',  ( -36.49999999999999289, -9.059673409587547965, 113.4689433211305811 ) ) ;
#11677=ORIENTED_EDGE ( 'NONE', *, *, #27495, .T. ) ;
#11721=EDGE_CURVE ( 'NONE', #12138, #26946, #26530, .T. ) ;
#11741=LINE ( 'NONE', #22188, #26991 ) ;
#11759=CARTESIAN_POINT ( 'NONE',  ( -37.49999999999999289, -15.63316754279159326, 121.0048025873809792 ) ) ;
#11794=DIRECTION ( 'NONE',  ( -1.000000000000000000, -0.000000000000000000, -0.000000000000000000 ) ) ;
#11809=EDGE_LOOP ( 'NONE', ( #3815, #7616, #11891, #18548 ) ) ;
#11838=DIRECTION ( 'NONE',  ( 1.000000000000000000, 0.000000000000000000, 0.000000000000000000 ) ) ;
#11875=ORIENTED_EDGE ( 'NONE', *, *, #20822, .F. ) ;
#11891=ORIENTED_EDGE ( 'NONE', *, *, #4438, .T. ) ;
#11987=DIRECTION ( 'NONE',  ( 1.000000000000000000, 0.000000000000000000, 0.000000000000000000 ) ) ;
#12117=AXIS2_PLACEMENT_3D ( 'NONE', #2140, #29133, #34535 ) ;
#12135=ORIENTED_EDGE ( 'NONE', *, *, #27500, .T. ) ;
#12138=VERTEX_POINT ( 'NONE', #13357 ) ;
#12186=CARTESIAN_POINT ( 'NONE',  ( -37.49999999999999289, -11.24969279549607748, 111.5585998451919778 ) ) ;
#12198=ORIENTED_EDGE ( 'NONE', *, *, #34763, .T. ) ;
#12297=CARTESIAN_POINT ( 'NONE',  ( -37.49999999999999289, -11.52052244843579309, 118.1848168619253556 ) ) ;
#12317=ORIENTED_EDGE ( 'NONE', *, *, #5289, .T. ) ;
#12347=DIRECTION ( 'NONE',  ( -0.000000000000000000, -0.7535859266250379829, -0.6573494133204068612 ) ) ;
#12369=CARTESIAN_POINT ( 'NONE',  ( -39.49999999999999289, -1.338792908815551458E-14, 114.0000000000000000 ) ) ;
#12400=ORIENTED_EDGE ( 'NONE', *, *, #5952, .F. ) ;
#12439=VERTEX_POINT ( 'NONE', #10741 ) ;
#12443=FACE_OUTER_BOUND ( 'NONE', #19328, .T. ) ;
#12560=DIRECTION ( 'NONE',  ( -1.000000000000000000, -0.000000000000000000, -0.000000000000000000 ) ) ;
#12579=ORIENTED_EDGE ( 'NONE', *, *, #4454, .F. ) ;
#12598=DIRECTION ( 'NONE',  ( -1.000000000000000000, -0.000000000000000000, -0.000000000000000000 ) ) ;
#12645=DIRECTION ( 'NONE',  ( 1.000000000000000000, 0.000000000000000000, -0.000000000000000000 ) ) ;
#12648=AXIS2_PLACEMENT_3D ( 'NONE', #32719, #476, #16310 ) ;
#12665=DIRECTION ( 'NONE',  ( 1.000000000000000000, 0.000000000000000000, 0.000000000000000000 ) ) ;
#12725=DIRECTION ( 'NONE',  ( 0.000000000000000000, 0.000000000000000000, 1.000000000000000000 ) ) ;
#12727=EDGE_LOOP ( 'NONE', ( #28179, #26141, #22339, #13080 ) ) ;
#12779=CIRCLE ( 'NONE', #32905, 9.999999999999994671 ) ;
#12814=VERTEX_POINT ( 'NONE', #25005 ) ;
#12841=LINE ( 'NONE', #12297, #22580 ) ;
#12893=CARTESIAN_POINT ( 'NONE',  ( -39.49999999999999289, -14.17619866229204106, 93.62476896299857287 ) ) ;
#12899=LINE ( 'NONE', #7834, #10505 ) ;
#12948=ORIENTED_EDGE ( 'NONE', *, *, #19490, .T. ) ;
#13073=CARTESIAN_POINT ( 'NONE',  ( -39.49999999999999289, -14.17619866229204106, 94.12476896299857287 ) ) ;
#13078=CARTESIAN_POINT ( 'NONE',  ( -39.49999999999999289, 0.4463568765849662556, 113.0433323525902125 ) ) ;
#13080=ORIENTED_EDGE ( 'NONE', *, *, #21096, .T. ) ;
#13089=ORIENTED_EDGE ( 'NONE', *, *, #21096, .F. ) ;
#13097=ADVANCED_FACE ( 'NONE', ( #1948 ), #26789, .T. ) ;
#13123=VERTEX_POINT ( 'NONE', #15423 ) ;
#13129=VERTEX_POINT ( 'NONE', #18315 ) ;
#13140=ORIENTED_EDGE ( 'NONE', *, *, #27073, .F. ) ;
#13216=VERTEX_POINT ( 'NONE', #30377 ) ;
#13270=EDGE_LOOP ( 'NONE', ( #4844, #9947, #34951, #27783 ) ) ;
#13285=CARTESIAN_POINT ( 'NONE',  ( -39.49999999999999289, -5.633167542791597704, 143.9590043477703887 ) ) ;
#13302=CARTESIAN_POINT ( 'NONE',  ( -39.49999999999999289, -5.633167542791597704, 121.0048025873810218 ) ) ;
#13357=CARTESIAN_POINT ( 'NONE',  ( -39.49999999999999289, -5.633167542791597704, 143.9590043477703887 ) ) ;
#13404=VECTOR ( 'NONE', #1146, 1000.000000000000000 ) ;
#13436=CARTESIAN_POINT ( 'NONE',  ( -36.49999999999999289, -11.52052244843579309, 118.1848168619253556 ) ) ;
#13468=ORIENTED_EDGE ( 'NONE', *, *, #7341, .F. ) ;
#13470=SURFACE_STYLE_USAGE ( .BOTH. , #2501 ) ;
#13584=CYLINDRICAL_SURFACE ( 'NONE', #3058, 0.5000000000000004441 ) ;
#13597=ORIENTED_EDGE ( 'NONE', *, *, #15368, .F. ) ;
#13659=CIRCLE ( 'NONE', #32621, 0.5000000000000004441 ) ;
#13768=FACE_OUTER_BOUND ( 'NONE', #10524, .T. ) ;
#13929=UNCERTAINTY_MEASURE_WITH_UNIT (LENGTH_MEASURE( 1.000000000000000082E-05 ), #15783, 'distance_accuracy_value', 'NONE');
#13992=EDGE_LOOP ( 'NONE', ( #34190, #24416, #20586, #26632 ) ) ;
#14031=DIRECTION ( 'NONE',  ( 0.000000000000000000, 0.000000000000000000, -1.000000000000000000 ) ) ;
#14078=VERTEX_POINT ( 'NONE', #19382 ) ;
#14085=EDGE_LOOP ( 'NONE', ( #31718, #24320, #31171, #29042 ) ) ;
#14099=DIRECTION ( 'NONE',  ( 0.000000000000000000, 0.000000000000000000, -1.000000000000000000 ) ) ;
#14101=DIRECTION ( 'NONE',  ( 0.000000000000000000, 0.000000000000000000, -1.000000000000000000 ) ) ;
#14146=CARTESIAN_POINT ( 'NONE',  ( -34.49999999999998579, -3.734562119078923992, 144.3977620171895637 ) ) ;
#14167=AXIS2_PLACEMENT_3D ( 'NONE', #33557, #8886, #22216 ) ;
#14195=DIRECTION ( 'NONE',  ( -0.000000000000000000, 0.7535859266250379829, 0.6573494133204068612 ) ) ;
#14269=VECTOR ( 'NONE', #29504, 1000.000000000000000 ) ;
#14327=CARTESIAN_POINT ( 'NONE',  ( -39.49999999999999289, 9.432411113711806294, 117.4309090467819772 ) ) ;
#14363=CYLINDRICAL_SURFACE ( 'NONE', #31310, 9.999999999999994671 ) ;
#14392=VERTEX_POINT ( 'NONE', #12893 ) ;
#14422=ORIENTED_EDGE ( 'NONE', *, *, #19082, .T. ) ;
#14468=( LENGTH_UNIT ( ) NAMED_UNIT ( * ) SI_UNIT ( .MILLI., .METRE. ) );
#14595=EDGE_CURVE ( 'NONE', #25789, #7877, #22206, .T. ) ;
#14606=CARTESIAN_POINT ( 'NONE',  ( -37.49999999999999289, -10.15468310254180651, 112.5137715831613008 ) ) ;
#14628=DIRECTION ( 'NONE',  ( 1.000000000000000000, 0.000000000000000000, 0.000000000000000000 ) ) ;
#14738=EDGE_CURVE ( 'NONE', #15547, #16117, #20204, .T. ) ;
#14750=VECTOR ( 'NONE', #22172, 1000.000000000000000 ) ;
#14812=EDGE_CURVE ( 'NONE', #17844, #20597, #27248, .T. ) ;
#14840=DIRECTION ( 'NONE',  ( -1.000000000000000000, -0.000000000000000000, -0.000000000000000000 ) ) ;
#14858=CYLINDRICAL_SURFACE ( 'NONE', #7762, 2.999999999999988898 ) ;
#14992=CARTESIAN_POINT ( 'NONE',  ( -37.49999999999999289, -11.52052244843579309, 115.1848168619253698 ) ) ;
#15003=EDGE_CURVE ( 'NONE', #26946, #25789, #3290, .T. ) ;
#15011=AXIS2_PLACEMENT_3D ( 'NONE', #33651, #30782, #6115 ) ;
#15018=EDGE_CURVE ( 'NONE', #33791, #25789, #21822, .T. ) ;
#15088=ORIENTED_EDGE ( 'NONE', *, *, #33049, .F. ) ;
#15115=CARTESIAN_POINT ( 'NONE',  ( -34.49999999999998579, -5.633167542791597704, 121.0048025873810218 ) ) ;
#15119=DIRECTION ( 'NONE',  ( 0.000000000000000000, 0.000000000000000000, -1.000000000000000000 ) ) ;
#15165=DIRECTION ( 'NONE',  ( 0.000000000000000000, 0.000000000000000000, -1.000000000000000000 ) ) ;
#15224=AXIS2_PLACEMENT_3D ( 'NONE', #25682, #20604, #9456 ) ;
#15258=EDGE_CURVE ( 'NONE', #11298, #26946, #26138, .T. ) ;
#15368=EDGE_CURVE ( 'NONE', #26302, #15547, #33883, .T. ) ;
#15423=CARTESIAN_POINT ( 'NONE',  ( -34.49999999999998579, -3.784235812937200460, 96.08311962715481513 ) ) ;
#15468=CARTESIAN_POINT ( 'NONE',  ( -37.49999999999999289, -11.52052244843579309, 115.1848168619253698 ) ) ;
#15535=EDGE_CURVE ( 'NONE', #13123, #12814, #5773, .T. ) ;
#15547=VERTEX_POINT ( 'NONE', #22317 ) ;
#15554=LINE ( 'NONE', #4087, #27990 ) ;
#15560=CARTESIAN_POINT ( 'NONE',  ( -39.49999999999999289, -15.63316754279159326, 121.0048025873809792 ) ) ;
#15582=ORIENTED_EDGE ( 'NONE', *, *, #34853, .F. ) ;
#15596=CARTESIAN_POINT ( 'NONE',  ( -39.49999999999999289, -4.676198662292047281, 104.0227405789415798 ) ) ;
#15600=LINE ( 'NONE', #15968, #25597 ) ;
#15630=CARTESIAN_POINT ( 'NONE',  ( -39.49999999999999289, 9.432411113711806294, 117.4309090467819772 ) ) ;
#15665=DIRECTION ( 'NONE',  ( -0.000000000000000000, -0.2588190451025194627, -0.9659258262890686453 ) ) ;
#15681=CARTESIAN_POINT ( 'NONE',  ( -39.49999999999999289, -14.17619866229204106, 94.12476896299857287 ) ) ;
#15684=DIRECTION ( 'NONE',  ( 1.000000000000000000, 0.000000000000000000, 0.000000000000000000 ) ) ;
#15711=EDGE_CURVE ( 'NONE', #11436, #5280, #10596, .T. ) ;
#15783=( LENGTH_UNIT ( ) NAMED_UNIT ( * ) SI_UNIT ( .MILLI., .METRE. ) );
#15968=CARTESIAN_POINT ( 'NONE',  ( -39.49999999999999289, -12.31102132296306451, 91.23752798680880005 ) ) ;
#16034=FACE_OUTER_BOUND ( 'NONE', #5715, .T. ) ;
#16072=DIRECTION ( 'NONE',  ( -1.000000000000000000, -0.000000000000000000, -0.000000000000000000 ) ) ;
#16102=DIRECTION ( 'NONE',  ( -0.000000000000000000, -0.7535859266250379829, -0.6573494133204068612 ) ) ;
#16117=VERTEX_POINT ( 'NONE', #10877 ) ;
#16142=ORIENTED_EDGE ( 'NONE', *, *, #20399, .T. ) ;
#16187=ORIENTED_EDGE ( 'NONE', *, *, #27086, .F. ) ;
#16191=ORIENTED_EDGE ( 'NONE', *, *, #16574, .F. ) ;
#16306=APPLICATION_CONTEXT ( 'automotive_design' ) ;
#16310=DIRECTION ( 'NONE',  ( 0.000000000000000000, 2.543449303551180694E-16, -1.000000000000000000 ) ) ;
#16342=EDGE_CURVE ( 'NONE', #26461, #23662, #3128, .T. ) ;
#16376=ORIENTED_EDGE ( 'NONE', *, *, #16342, .T. ) ;
#16469=VECTOR ( 'NONE', #9735, 1000.000000000000000 ) ;
#16493=CARTESIAN_POINT ( 'NONE',  ( -34.49999999999998579, -14.67619866229204284, 93.25874355921412473 ) ) ;
#16523=EDGE_CURVE ( 'NONE', #29235, #19887, #9701, .T. ) ;
#16525=PLANE ( 'NONE',  #2893 ) ;
#16574=EDGE_CURVE ( 'NONE', #26937, #15547, #3399, .T. ) ;
#16579=DIRECTION ( 'NONE',  ( 0.000000000000000000, 0.000000000000000000, -1.000000000000000000 ) ) ;
#16581=CARTESIAN_POINT ( 'NONE',  ( -39.49999999999999289, -1.387778780781445676E-14, 110.0000000000000000 ) ) ;
#16597=EDGE_CURVE ( 'NONE', #33309, #1785, #4600, .T. ) ;
#16600=CYLINDRICAL_SURFACE ( 'NONE', #7289, 1.000000000000000888 ) ;
#16718=ORIENTED_EDGE ( 'NONE', *, *, #14738, .F. ) ;
#16734=CARTESIAN_POINT ( 'NONE',  ( -34.49999999999998579, -1.387778780781445676E-14, 106.0000000000000000 ) ) ;
#16771=ORIENTED_EDGE ( 'NONE', *, *, #20399, .F. ) ;
#16819=ORIENTED_EDGE ( 'NONE', *, *, #16523, .F. ) ;
#16857=ORIENTED_EDGE ( 'NONE', *, *, #9253, .F. ) ;
#16992=VERTEX_POINT ( 'NONE', #3486 ) ;
#17002=EDGE_CURVE ( 'NONE', #32244, #4537, #11741, .T. ) ;
#17016=CARTESIAN_POINT ( 'NONE',  ( -36.49999999999999289, -11.52052244843579309, 115.1848168619253698 ) ) ;
#17022=CARTESIAN_POINT ( 'NONE',  ( -39.49999999999999289, -14.17619866229204106, 93.62476896299857287 ) ) ;
#17027=CIRCLE ( 'NONE', #5568, 2.999999999999988898 ) ;
#17049=AXIS2_PLACEMENT_3D ( 'NONE', #17411, #11838, #8957 ) ;
#17052=CARTESIAN_POINT ( 'NONE',  ( -34.49999999999998579, -5.633167542791597704, 121.0048025873810218 ) ) ;
#17072=ORIENTED_EDGE ( 'NONE', *, *, #35203, .F. ) ;
#17078=CYLINDRICAL_SURFACE ( 'NONE', #7927, 4.999999999999990230 ) ;
#17086=EDGE_LOOP ( 'NONE', ( #1392, #25636 ) ) ;
#17106=VECTOR ( 'NONE', #4332, 1000.000000000000000 ) ;
#17124=ORIENTED_EDGE ( 'NONE', *, *, #18754, .T. ) ;
#17216=CIRCLE ( 'NONE', #1153, 0.5000000000000004441 ) ;
#17222=CARTESIAN_POINT ( 'NONE',  ( -36.49999999999999289, -10.15468310254180651, 112.5137715831613008 ) ) ;
#17227=DIRECTION ( 'NONE',  ( 1.000000000000000000, 0.000000000000000000, 0.000000000000000000 ) ) ;
#17357=DIRECTION ( 'NONE',  ( 1.000000000000000000, 0.000000000000000000, 0.000000000000000000 ) ) ;
#17366=DIRECTION ( 'NONE',  ( 0.000000000000000000, 4.163336342344333240E-14, -1.000000000000000000 ) ) ;
#17381=ORIENTED_EDGE ( 'NONE', *, *, #16574, .T. ) ;
#17399=CARTESIAN_POINT ( 'NONE',  ( -39.49999999999999289, -5.633167542791597704, 121.0048025873810218 ) ) ;
#17406=ADVANCED_FACE ( 'NONE', ( #21564 ), #26649, .F. ) ;
#17411=CARTESIAN_POINT ( 'NONE',  ( -39.49999999999999289, 0.4463568765849662556, 113.0433323525902125 ) ) ;
#17453=LINE ( 'NONE', #1092, #22582 ) ;
#17475=ORIENTED_EDGE ( 'NONE', *, *, #24717, .F. ) ;
#17539=LINE ( 'NONE', #28194, #28383 ) ;
#17689=CARTESIAN_POINT ( 'NONE',  ( -39.49999999999999289, -12.31102132296306451, 91.73752798680880005 ) ) ;
#17713=ORIENTED_EDGE ( 'NONE', *, *, #10603, .F. ) ;
#17732=AXIS2_PLACEMENT_3D ( 'NONE', #9268, #14840, #1171 ) ;
#17776=ORIENTED_EDGE ( 'NONE', *, *, #25973, .F. ) ;
#17814=VERTEX_POINT ( 'NONE', #12369 ) ;
#17844=VERTEX_POINT ( 'NONE', #17399 ) ;
#17868=CARTESIAN_POINT ( 'NONE',  ( -39.49999999999999289, -1.338792908815551458E-14, 114.0000000000000000 ) ) ;
#17961=AXIS2_PLACEMENT_3D ( 'NONE', #15681, #33492, #16579 ) ;
#18000=ORIENTED_EDGE ( 'NONE', *, *, #21925, .F. ) ;
#18002=DIRECTION ( 'NONE',  ( 1.000000000000000000, 0.000000000000000000, 0.000000000000000000 ) ) ;
#18016=ORIENTED_EDGE ( 'NONE', *, *, #9265, .F. ) ;
#18040=AXIS2_PLACEMENT_3D ( 'NONE', #22950, #6930, #6394 ) ;
#18144=CIRCLE ( 'NONE', #33661, 9.999999999999994671 ) ;
#18292=DIRECTION ( 'NONE',  ( 1.000000000000000000, 0.000000000000000000, 0.000000000000000000 ) ) ;
#18315=CARTESIAN_POINT ( 'NONE',  ( -37.49999999999999289, -6.699660887819688604, 116.5112005972652014 ) ) ;
#18454=AXIS2_PLACEMENT_3D ( 'NONE', #20453, #12560, #9677 ) ;
#18499=DIRECTION ( 'NONE',  ( 0.000000000000000000, 0.000000000000000000, -1.000000000000000000 ) ) ;
#18506=VERTEX_POINT ( 'NONE', #5435 ) ;
#18548=ORIENTED_EDGE ( 'NONE', *, *, #21925, .T. ) ;
#18600=ORIENTED_EDGE ( 'NONE', *, *, #15368, .T. ) ;
#18647=ORIENTED_EDGE ( 'NONE', *, *, #23353, .T. ) ;
#18654=CARTESIAN_POINT ( 'NONE',  ( -39.49999999999999289, -3.784235812937200460, 96.08311962715481513 ) ) ;
#18754=EDGE_CURVE ( 'NONE', #26302, #26408, #1808, .T. ) ;
#18880=DIRECTION ( 'NONE',  ( 1.000000000000000000, 0.000000000000000000, 0.000000000000000000 ) ) ;
#18920=ORIENTED_EDGE ( 'NONE', *, *, #16597, .T. ) ;
#18987=EDGE_LOOP ( 'NONE', ( #18000, #15582 ) ) ;
#18998=DIRECTION ( 'NONE',  ( 0.000000000000000000, 0.8660254037844381525, 0.5000000000000006661 ) ) ;
#19082=EDGE_CURVE ( 'NONE', #10765, #26461, #20978, .T. ) ;
#19089=VERTEX_POINT ( 'NONE', #23158 ) ;
#19120=AXIS2_PLACEMENT_3D ( 'NONE', #5837, #25458, #14101 ) ;
#19180=AXIS2_PLACEMENT_3D ( 'NONE', #19573, #22630, #19227 ) ;
#19186=PLANE ( 'NONE',  #23546 ) ;
#19203=CARTESIAN_POINT ( 'NONE',  ( -36.49999999999999289, -11.52052244843579309, 115.1848168619253698 ) ) ;
#19218=AXIS2_PLACEMENT_3D ( 'NONE', #15468, #1100, #4342 ) ;
#19227=DIRECTION ( 'NONE',  ( 0.000000000000000000, -6.245004513516508695E-15, -1.000000000000000000 ) ) ;
#19239=VERTEX_POINT ( 'NONE', #13436 ) ;
#19259=VECTOR ( 'NONE', #19466, 1000.000000000000000 ) ;
#19268=CIRCLE ( 'NONE', #6599, 9.999999999999994671 ) ;
#19310=DIRECTION ( 'NONE',  ( 1.000000000000000000, 0.000000000000000000, 0.000000000000000000 ) ) ;
#19328=EDGE_LOOP ( 'NONE', ( #21180, #23377, #25893, #12579, #16142, #11875, #8713, #12135 ) ) ;
#19333=CARTESIAN_POINT ( 'NONE',  ( -37.49999999999999289, -11.24969279549607748, 111.5585998451919778 ) ) ;
#19344=SURFACE_STYLE_USAGE ( .BOTH. , #451 ) ;
#19382=CARTESIAN_POINT ( 'NONE',  ( -34.49999999999998579, -14.17619866229204106, 93.62476896299857287 ) ) ;
#19466=DIRECTION ( 'NONE',  ( 1.000000000000000000, 0.000000000000000000, 0.000000000000000000 ) ) ;
#19490=EDGE_CURVE ( 'NONE', #30962, #13123, #31628, .T. ) ;
#19526=CARTESIAN_POINT ( 'NONE',  ( -34.49999999999998579, -14.67619866229204284, 104.0227405789415371 ) ) ;
#19566=CARTESIAN_POINT ( 'NONE',  ( -39.49999999999999289, -14.67619866229204284, 93.25874355921412473 ) ) ;
#19573=CARTESIAN_POINT ( 'NONE',  ( -36.49999999999999289, -4.676198662292047281, 104.0227405789415798 ) ) ;
#19599=FACE_OUTER_BOUND ( 'NONE', #22009, .T. ) ;
#19611=EDGE_LOOP ( 'NONE', ( #5017, #20551, #17381, #13597, #17713, #2585, #18647, #1472, #30040, #28037, #21706, #11397, #1085, #26548, #25473, #17475 ) ) ;
#19639=CARTESIAN_POINT ( 'NONE',  ( -39.49999999999999289, -4.633167542791596816, 143.9590043477703887 ) ) ;
#19665=FACE_OUTER_BOUND ( 'NONE', #11809, .T. ) ;
#19706=ADVANCED_FACE ( 'NONE', ( #10922, #21517 ), #19186, .F. ) ;
#19729=ORIENTED_EDGE ( 'NONE', *, *, #4438, .F. ) ;
#19750=ADVANCED_FACE ( 'NONE', ( #2127 ), #24087, .T. ) ;
#19769=DIRECTION ( 'NONE',  ( 0.000000000000000000, 0.7535859266250380939, 0.6573494133204066392 ) ) ;
#19770=CYLINDRICAL_SURFACE ( 'NONE', #15011, 0.5000000000000004441 ) ;
#19788=VECTOR ( 'NONE', #14195, 1000.000000000000000 ) ;
#19789=ORIENTED_EDGE ( 'NONE', *, *, #14595, .T. ) ;
#19808=DIRECTION ( 'NONE',  ( 1.000000000000000000, 0.000000000000000000, 0.000000000000000000 ) ) ;
#19853=CARTESIAN_POINT ( 'NONE',  ( -39.49999999999999289, -14.67619866229204284, 104.0227405789415371 ) ) ;
#19879=CARTESIAN_POINT ( 'NONE',  ( -39.49999999999999289, -11.24969279549607748, 111.5585998451919778 ) ) ;
#19880=CIRCLE ( 'NONE', #34892, 4.999999999999990230 ) ;
#19887=VERTEX_POINT ( 'NONE', #19526 ) ;
#20042=ORIENTED_EDGE ( 'NONE', *, *, #15018, .T. ) ;
#20101=DIRECTION ( 'NONE',  ( 0.000000000000000000, 0.000000000000000000, -1.000000000000000000 ) ) ;
#20128=ORIENTED_EDGE ( 'NONE', *, *, #14595, .F. ) ;
#20191=DIRECTION ( 'NONE',  ( 0.000000000000000000, 0.000000000000000000, -1.000000000000000000 ) ) ;
#20204=LINE ( 'NONE', #6905, #1529 ) ;
#20272=EDGE_CURVE ( 'NONE', #30962, #26405, #32472, .T. ) ;
#20334=CARTESIAN_POINT ( 'NONE',  ( -39.49999999999999289, 7.019851009788996343, 105.5074730863398003 ) ) ;
#20359=CARTESIAN_POINT ( 'NONE',  ( -36.49999999999999289, -6.699660887819688604, 116.5112005972652014 ) ) ;
#20391=ORIENTED_EDGE ( 'NONE', *, *, #27489, .T. ) ;
#20394=CARTESIAN_POINT ( 'NONE',  ( -39.49999999999999289, -14.67619866229204284, 93.25874355921412473 ) ) ;
#20399=EDGE_CURVE ( 'NONE', #5280, #5287, #27798, .T. ) ;
#20453=CARTESIAN_POINT ( 'NONE',  ( -34.49999999999998579, -15.63316754279159326, 121.0048025873809792 ) ) ;
#20477=ORIENTED_EDGE ( 'NONE', *, *, #15711, .F. ) ;
#20479=EDGE_LOOP ( 'NONE', ( #27910, #3767, #5771, #17124 ) ) ;
#20480=CIRCLE ( 'NONE', #6700, 4.000000000000003553 ) ;
#20487=ADVANCED_FACE ( 'NONE', ( #2179 ), #4524, .T. ) ;
#20493=VERTEX_POINT ( 'NONE', #20359 ) ;
#20507=CARTESIAN_POINT ( 'NONE',  ( -39.49999999999999289, -12.00833024919777081, 94.79903810567661537 ) ) ;
#20512=VECTOR ( 'NONE', #6329, 1000.000000000000000 ) ;
#20550=EDGE_CURVE ( 'NONE', #19239, #19089, #22450, .T. ) ;
#20551=ORIENTED_EDGE ( 'NONE', *, *, #9265, .T. ) ;
#20565=DIRECTION ( 'NONE',  ( 0.000000000000000000, 0.000000000000000000, -1.000000000000000000 ) ) ;
#20571=DIRECTION ( 'NONE',  ( -0.000000000000000000, -0.2588190451025194627, -0.9659258262890686453 ) ) ;
#20577=CARTESIAN_POINT ( 'NONE',  ( -37.49999999999999289, -11.52052244843579309, 115.1848168619253698 ) ) ;
#20586=ORIENTED_EDGE ( 'NONE', *, *, #20550, .T. ) ;
#20597=VERTEX_POINT ( 'NONE', #17052 ) ;
#20604=DIRECTION ( 'NONE',  ( 1.000000000000000000, 0.000000000000000000, 0.000000000000000000 ) ) ;
#20609=DIRECTION ( 'NONE',  ( -1.000000000000000000, -0.000000000000000000, -0.000000000000000000 ) ) ;
#20655=CARTESIAN_POINT ( 'NONE',  ( -39.49999999999999289, -14.67619866229204284, 94.12476896299857287 ) ) ;
#20710=CARTESIAN_POINT ( 'NONE',  ( -39.49999999999999289, 9.432411113711806294, 117.4309090467819772 ) ) ;
#20719=PRODUCT ( 'Heavy-Duty Locking Pawl', 'Heavy-Duty Locking Pawl', '', ( #33984 ) ) ;
#20726=AXIS2_PLACEMENT_3D ( 'NONE', #850, #17227, #20101 ) ;
#20822=EDGE_CURVE ( 'NONE', #20597, #5287, #8683, .T. ) ;
#20957=DIRECTION ( 'NONE',  ( 1.000000000000000000, 0.000000000000000000, 0.000000000000000000 ) ) ;
#20969=CARTESIAN_POINT ( 'NONE',  ( -39.49999999999999289, -13.10640646055107084, 90.70096189432331357 ) ) ;
#20970=ORIENTED_EDGE ( 'NONE', *, *, #22491, .T. ) ;
#20978=LINE ( 'NONE', #12186, #30951 ) ;
#21042=AXIS2_PLACEMENT_3D ( 'NONE', #29580, #15684, #34991 ) ;
#21096=EDGE_CURVE ( 'NONE', #6914, #12814, #6393, .T. ) ;
#21108=ORIENTED_EDGE ( 'NONE', *, *, #34839, .F. ) ;
#21109=DIRECTION ( 'NONE',  ( 1.000000000000000000, 0.000000000000000000, 0.000000000000000000 ) ) ;
#21180=ORIENTED_EDGE ( 'NONE', *, *, #26055, .T. ) ;
#21259=ORIENTED_EDGE ( 'NONE', *, *, #5772, .F. ) ;
#21307=AXIS2_PLACEMENT_3D ( 'NONE', #26589, #12725, #18292 ) ;
#21315=EDGE_LOOP ( 'NONE', ( #5819, #10179, #24687, #6272, #30311, #16819, #29196, #35312 ) ) ;
#21367=DIRECTION ( 'NONE',  ( 1.000000000000000000, 0.000000000000000000, -0.000000000000000000 ) ) ;
#21449=VECTOR ( 'NONE', #11987, 1000.000000000000000 ) ;
#21456=VECTOR ( 'NONE', #4216, 1000.000000000000000 ) ;
#21517=FACE_OUTER_BOUND ( 'NONE', #19611, .T. ) ;
#21543=CARTESIAN_POINT ( 'NONE',  ( -34.49999999999998579, -13.92619866229204106, 93.69175626110634880 ) ) ;
#21564=FACE_OUTER_BOUND ( 'NONE', #32289, .T. ) ;
#21632=VECTOR ( 'NONE', #25951, 1000.000000000000000 ) ;
#21706=ORIENTED_EDGE ( 'NONE', *, *, #27500, .F. ) ;
#21717=DIRECTION ( 'NONE',  ( -1.000000000000000000, -0.000000000000000000, -0.000000000000000000 ) ) ;
#21731=EDGE_LOOP ( 'NONE', ( #18920, #3760, #17072, #9508 ) ) ;
#21750=CARTESIAN_POINT ( 'NONE',  ( -37.49999999999999289, -11.52052244843579309, 115.1848168619253698 ) ) ;
#21822=LINE ( 'NONE', #25062, #7874 ) ;
#21859=CARTESIAN_POINT ( 'NONE',  ( -39.49999999999999289, -12.31102132296306451, 91.73752798680880005 ) ) ;
#21876=VECTOR ( 'NONE', #19310, 1000.000000000000000 ) ;
#21925=EDGE_CURVE ( 'NONE', #31088, #16992, #935, .T. ) ;
#22009=EDGE_LOOP ( 'NONE', ( #12198, #23341, #25110, #733 ) ) ;
#22016=PRODUCT_DEFINITION_CONTEXT ( 'detailed design', #16306, 'design' ) ;
#22042=DIRECTION ( 'NONE',  ( 0.000000000000000000, 0.000000000000000000, -1.000000000000000000 ) ) ;
#22061=AXIS2_PLACEMENT_3D ( 'NONE', #23426, #29202, #15119 ) ;
#22080=LINE ( 'NONE', #16493, #6128 ) ;
#22156=AXIS2_PLACEMENT_3D ( 'NONE', #9651, #10002, #29280 ) ;
#22172=DIRECTION ( 'NONE',  ( 1.000000000000000000, 0.000000000000000000, 0.000000000000000000 ) ) ;
#22188=CARTESIAN_POINT ( 'NONE',  ( -36.99999999999999289, -12.47865190846804495, 110.2774766518096925 ) ) ;
#22206=CIRCLE ( 'NONE', #14167, 1.000000000000000888 ) ;
#22216=DIRECTION ( 'NONE',  ( 0.000000000000000000, 0.000000000000000000, -1.000000000000000000 ) ) ;
#22227=( NAMED_UNIT ( * ) PLANE_ANGLE_UNIT ( ) SI_UNIT ( $, .RADIAN. ) );
#22317=CARTESIAN_POINT ( 'NONE',  ( -39.49999999999999289, -12.79398423610758684, 91.86693750936007064 ) ) ;
#22339=ORIENTED_EDGE ( 'NONE', *, *, #24717, .T. ) ;
#22352=EDGE_LOOP ( 'NONE', ( #2423, #8991, #12317, #6960, #7426, #35525, #23975 ) ) ;
#22398=SURFACE_STYLE_FILL_AREA ( #25121 ) ;
#22441=FACE_OUTER_BOUND ( 'NONE', #20479, .T. ) ;
#22450=CIRCLE ( 'NONE', #20726, 2.999999999999988898 ) ;
#22491=EDGE_CURVE ( 'NONE', #31548, #10765, #22955, .T. ) ;
#22508=DIRECTION ( 'NONE',  ( 0.000000000000000000, 0.7535859266250380939, 0.6573494133204066392 ) ) ;
#22523=CARTESIAN_POINT ( 'NONE',  ( -39.49999999999999289, -3.734562119078910225, 144.3977620171895637 ) ) ;
#22580=VECTOR ( 'NONE', #12665, 1000.000000000000000 ) ;
#22582=VECTOR ( 'NONE', #6837, 1000.000000000000000 ) ;
#22616=DIRECTION ( 'NONE',  ( 0.000000000000000000, -0.7535859266250379829, -0.6573494133204068612 ) ) ;
#22630=DIRECTION ( 'NONE',  ( -1.000000000000000000, -0.000000000000000000, -0.000000000000000000 ) ) ;
#22636=CARTESIAN_POINT ( 'NONE',  ( -36.49999999999999289, -11.24969279549607748, 111.5585998451919778 ) ) ;
#22662=FACE_OUTER_BOUND ( 'NONE', #33260, .T. ) ;
#22680=VECTOR ( 'NONE', #11498, 1000.000000000000000 ) ;
#22777=CIRCLE ( 'NONE', #4434, 0.5000000000000004441 ) ;
#22811=CARTESIAN_POINT ( 'NONE',  ( -39.49999999999999289, -4.633167542791596816, 143.9590043477703887 ) ) ;
#22884=STYLED_ITEM ( 'NONE', ( #32539 ), #33931 ) ;
#22907=EDGE_CURVE ( 'NONE', #12814, #33791, #12779, .T. ) ;
#22950=CARTESIAN_POINT ( 'NONE',  ( -36.49999999999999289, -15.63316754279159326, 121.0048025873809792 ) ) ;
#22955=LINE ( 'NONE', #19879, #21449 ) ;
#23088=DIRECTION ( 'NONE',  ( 1.000000000000000000, 0.000000000000000000, 0.000000000000000000 ) ) ;
#23158=CARTESIAN_POINT ( 'NONE',  ( -36.49999999999999289, -11.52052244843579309, 112.1848168619253840 ) ) ;
#23277=ORIENTED_EDGE ( 'NONE', *, *, #25698, .T. ) ;
#23303=PRODUCT_DEFINITION_SHAPE ( 'NONE', 'NONE',  #30188 ) ;
#23315=DIRECTION ( 'NONE',  ( 0.000000000000000000, 0.000000000000000000, -1.000000000000000000 ) ) ;
#23341=ORIENTED_EDGE ( 'NONE', *, *, #17002, .T. ) ;
#23353=EDGE_CURVE ( 'NONE', #14392, #1785, #9375, .T. ) ;
#23377=ORIENTED_EDGE ( 'NONE', *, *, #6366, .T. ) ;
#23426=CARTESIAN_POINT ( 'NONE',  ( -39.49999999999999289, -15.63316754279159326, 121.0048025873809792 ) ) ;
#23513=ORIENTED_EDGE ( 'NONE', *, *, #5952, .T. ) ;
#23546=AXIS2_PLACEMENT_3D ( 'NONE', #5177, #26779, #2474 ) ;
#23557=ORIENTED_EDGE ( 'NONE', *, *, #7227, .F. ) ;
#23615=DIRECTION ( 'NONE',  ( 0.000000000000000000, -0.4387576694191721027, 0.8986054237126862576 ) ) ;
#23662=VERTEX_POINT ( 'NONE', #17222 ) ;
#23691=DIRECTION ( 'NONE',  ( 1.000000000000000000, 0.000000000000000000, 0.000000000000000000 ) ) ;
#23786=CYLINDRICAL_SURFACE ( 'NONE', #22061, 9.999999999999994671 ) ;
#23827=DIRECTION ( 'NONE',  ( 1.000000000000000000, 0.000000000000000000, 0.000000000000000000 ) ) ;
#23895=AXIS2_PLACEMENT_3D ( 'NONE', #17016, #28025, #35606 ) ;
#23975=ORIENTED_EDGE ( 'NONE', *, *, #4454, .T. ) ;
#24010=AXIS2_PLACEMENT_3D ( 'NONE', #11074, #7824, #22042 ) ;
#24019=CARTESIAN_POINT ( 'NONE',  ( -39.49999999999999289, -5.633167542791597704, 121.0048025873810218 ) ) ;
#24038=CARTESIAN_POINT ( 'NONE',  ( -37.49999999999999289, -12.47865190846804495, 110.2774766518096925 ) ) ;
#24087=PLANE ( 'NONE',  #6275 ) ;
#24151=ORIENTED_EDGE ( 'NONE', *, *, #26055, .F. ) ;
#24195=EDGE_CURVE ( 'NONE', #20493, #4537, #9994, .T. ) ;
#24221=ORIENTED_EDGE ( 'NONE', *, *, #19490, .F. ) ;
#24226=LINE ( 'NONE', #29276, #8078 ) ;
#24247=ADVANCED_FACE ( 'NONE', ( #6708 ), #9770, .T. ) ;
#24275=CARTESIAN_POINT ( 'NONE',  ( -39.49999999999999289, -3.734562119078923992, 144.3977620171895637 ) ) ;
#24320=ORIENTED_EDGE ( 'NONE', *, *, #5249, .T. ) ;
#24363=DIRECTION ( 'NONE',  ( 1.000000000000000000, 0.000000000000000000, 0.000000000000000000 ) ) ;
#24395=FACE_OUTER_BOUND ( 'NONE', #28029, .T. ) ;
#24416=ORIENTED_EDGE ( 'NONE', *, *, #702, .T. ) ;
#24444=CARTESIAN_POINT ( 'NONE',  ( -39.49999999999999289, -14.67619866229204284, 104.0227405789415371 ) ) ;
#24451=CARTESIAN_POINT ( 'NONE',  ( -39.49999999999999289, -3.784235812937200460, 96.08311962715481513 ) ) ;
#24609=DIRECTION ( 'NONE',  ( 0.000000000000000000, 0.6573494133204066392, -0.7535859266250380939 ) ) ;
#24667=ORIENTED_EDGE ( 'NONE', *, *, #6366, .F. ) ;
#24687=ORIENTED_EDGE ( 'NONE', *, *, #22491, .F. ) ;
#24701=EDGE_CURVE ( 'NONE', #1785, #34547, #25234, .T. ) ;
#24717=EDGE_CURVE ( 'NONE', #1934, #6914, #3275, .T. ) ;
#24728=PRODUCT_DEFINITION_FORMATION_WITH_SPECIFIED_SOURCE ( 'ANY', '', #20719, .NOT_KNOWN. ) ;
#24803=DIRECTION ( 'NONE',  ( 1.000000000000000000, 0.000000000000000000, 0.000000000000000000 ) ) ;
#24836=DIRECTION ( 'NONE',  ( 0.000000000000000000, 0.000000000000000000, -1.000000000000000000 ) ) ;
#24920=DIRECTION ( 'NONE',  ( 1.000000000000000000, 0.000000000000000000, 0.000000000000000000 ) ) ;
#24947=( NAMED_UNIT ( * ) SI_UNIT ( $, .STERADIAN. ) SOLID_ANGLE_UNIT ( ) );
#24976=DIRECTION ( 'NONE',  ( 0.000000000000000000, 0.000000000000000000, -1.000000000000000000 ) ) ;
#24989=FACE_OUTER_BOUND ( 'NONE', #2670, .T. ) ;
#24991=ORIENTED_EDGE ( 'NONE', *, *, #23353, .F. ) ;
#25005=CARTESIAN_POINT ( 'NONE',  ( -34.49999999999998579, 7.019851009788996343, 105.5074730863398003 ) ) ;
#25062=CARTESIAN_POINT ( 'NONE',  ( -34.49999999999998579, 9.432411113711806294, 117.4309090467819772 ) ) ;
#25110=ORIENTED_EDGE ( 'NONE', *, *, #24195, .F. ) ;
#25121=FILL_AREA_STYLE ('',( #28346 ) ) ;
#25156=LINE ( 'NONE', #17022, #411 ) ;
#25161=VECTOR ( 'NONE', #15665, 1000.000000000000000 ) ;
#25197=LINE ( 'NONE', #22636, #19788 ) ;
#25229=DIRECTION ( 'NONE',  ( 0.000000000000000000, 0.000000000000000000, -1.000000000000000000 ) ) ;
#25234=LINE ( 'NONE', #33157, #19259 ) ;
#25317=DIRECTION ( 'NONE',  ( 1.000000000000000000, 0.000000000000000000, 0.000000000000000000 ) ) ;
#25458=DIRECTION ( 'NONE',  ( 1.000000000000000000, 0.000000000000000000, 0.000000000000000000 ) ) ;
#25473=ORIENTED_EDGE ( 'NONE', *, *, #8778, .F. ) ;
#25493=ORIENTED_EDGE ( 'NONE', *, *, #14812, .T. ) ;
#25547=DIRECTION ( 'NONE',  ( 1.000000000000000000, 0.000000000000000000, 0.000000000000000000 ) ) ;
#25597=VECTOR ( 'NONE', #26623, 1000.000000000000000 ) ;
#25636=ORIENTED_EDGE ( 'NONE', *, *, #34839, .T. ) ;
#25651=CARTESIAN_POINT ( 'NONE',  ( -39.49999999999999289, -1.387778780781445676E-14, 110.0000000000000000 ) ) ;
#25657=PRESENTATION_STYLE_ASSIGNMENT (( #19344 ) ) ;
#25682=CARTESIAN_POINT ( 'NONE',  ( -34.49999999999998579, -14.17619866229204106, 94.12476896299857287 ) ) ;
#25698=EDGE_CURVE ( 'NONE', #16117, #34424, #2691, .T. ) ;
#25789=VERTEX_POINT ( 'NONE', #14146 ) ;
#25834=AXIS2_PLACEMENT_3D ( 'NONE', #6875, #12645, #1475 ) ;
#25893=ORIENTED_EDGE ( 'NONE', *, *, #666, .F. ) ;
#25951=DIRECTION ( 'NONE',  ( 1.000000000000000000, 0.000000000000000000, 0.000000000000000000 ) ) ;
#25960=APPLICATION_CONTEXT ( 'automotive_design' ) ;
#25973=EDGE_CURVE ( 'NONE', #18506, #14392, #22777, .T. ) ;
#25986=DIRECTION ( 'NONE',  ( 1.000000000000000000, 0.000000000000000000, 0.000000000000000000 ) ) ;
#26055=EDGE_CURVE ( 'NONE', #8765, #11436, #15554, .T. ) ;
#26063=ORIENTED_EDGE ( 'NONE', *, *, #11721, .F. ) ;
#26103=CIRCLE ( 'NONE', #18040, 9.999999999999994671 ) ;
#26138=LINE ( 'NONE', #20710, #4487 ) ;
#26141=ORIENTED_EDGE ( 'NONE', *, *, #7009, .F. ) ;
#26163=DIRECTION ( 'NONE',  ( 0.000000000000000000, 0.000000000000000000, -1.000000000000000000 ) ) ;
#26302=VERTEX_POINT ( 'NONE', #8532 ) ;
#26405=VERTEX_POINT ( 'NONE', #968 ) ;
#26408=VERTEX_POINT ( 'NONE', #27813 ) ;
#26461=VERTEX_POINT ( 'NONE', #26847 ) ;
#26530=CIRCLE ( 'NONE', #5827, 1.000000000000000888 ) ;
#26548=ORIENTED_EDGE ( 'NONE', *, *, #15258, .F. ) ;
#26589=CARTESIAN_POINT ( 'NONE',  ( 0.000000000000000000, 0.000000000000000000, 0.000000000000000000 ) ) ;
#26623=DIRECTION ( 'NONE',  ( 1.000000000000000000, 0.000000000000000000, 0.000000000000000000 ) ) ;
#26632=ORIENTED_EDGE ( 'NONE', *, *, #5249, .F. ) ;
#26649=PLANE ( 'NONE',  #28724 ) ;
#26752=DIRECTION ( 'NONE',  ( 0.000000000000000000, 4.163336342344333240E-14, -1.000000000000000000 ) ) ;
#26779=DIRECTION ( 'NONE',  ( 1.000000000000000000, 0.000000000000000000, 0.000000000000000000 ) ) ;
#26789=PLANE ( 'NONE',  #12117 ) ;
#26798=CARTESIAN_POINT ( 'NONE',  ( -39.49999999999999289, -12.31102132296306451, 91.23752798680880005 ) ) ;
#26847=CARTESIAN_POINT ( 'NONE',  ( -37.49999999999999289, -10.15468310254180651, 112.5137715831613008 ) ) ;
#26937=VERTEX_POINT ( 'NONE', #26798 ) ;
#26946=VERTEX_POINT ( 'NONE', #24275 ) ;
#26991=VECTOR ( 'NONE', #33188, 1000.000000000000000 ) ;
#27024=AXIS2_PLACEMENT_3D ( 'NONE', #34567, #29169, #1434 ) ;
#27073=EDGE_CURVE ( 'NONE', #26937, #34424, #15600, .T. ) ;
#27086=EDGE_CURVE ( 'NONE', #34424, #30962, #3186, .T. ) ;
#27144=AXIS2_PLACEMENT_3D ( 'NONE', #8588, #11131, #22616 ) ;
#27164=EDGE_CURVE ( 'NONE', #33309, #19887, #30550, .T. ) ;
#27241=ORIENTED_EDGE ( 'NONE', *, *, #34853, .T. ) ;
#27248=LINE ( 'NONE', #24019, #27430 ) ;
#27343=VECTOR ( 'NONE', #12347, 1000.000000000000000 ) ;
#27405=ADVANCED_FACE ( 'NONE', ( #7644 ), #4263, .T. ) ;
#27430=VECTOR ( 'NONE', #24363, 1000.000000000000000 ) ;
#27433=EDGE_LOOP ( 'NONE', ( #11572, #23277, #11634, #12948, #30921, #11380, #20042, #19789, #6668, #32863, #20391, #6029, #30287, #9033, #23513, #7915 ) ) ;
#27476=ORIENTED_EDGE ( 'NONE', *, *, #7341, .T. ) ;
#27489=EDGE_CURVE ( 'NONE', #5287, #29235, #29455, .T. ) ;
#27495=EDGE_CURVE ( 'NONE', #28348, #13216, #8355, .T. ) ;
#27500=EDGE_CURVE ( 'NONE', #17844, #8765, #28494, .T. ) ;
#27553=VECTOR ( 'NONE', #9488, 1000.000000000000227 ) ;
#27783=ORIENTED_EDGE ( 'NONE', *, *, #7362, .F. ) ;
#27798=LINE ( 'NONE', #3134, #21876 ) ;
#27809=CARTESIAN_POINT ( 'NONE',  ( -34.49999999999998579, 0.4463568765849662556, 113.0433323525902125 ) ) ;
#27813=CARTESIAN_POINT ( 'NONE',  ( -34.49999999999998579, -12.00833024919777081, 94.79903810567661537 ) ) ;
#27864=CARTESIAN_POINT ( 'NONE',  ( -39.49999999999999289, -11.24969279549607748, 111.5585998451919778 ) ) ;
#27903=DIRECTION ( 'NONE',  ( 1.000000000000000000, 0.000000000000000000, 0.000000000000000000 ) ) ;
#27910=ORIENTED_EDGE ( 'NONE', *, *, #28625, .F. ) ;
#27983=CARTESIAN_POINT ( 'NONE',  ( -34.49999999999998579, -11.24969279549607748, 111.5585998451919778 ) ) ;
#27990=VECTOR ( 'NONE', #20957, 1000.000000000000000 ) ;
#27998=SHAPE_REPRESENTATION_RELATIONSHIP ( 'NONE' , 'NONE' ,  #33958, #3950 ) ;
#28025=DIRECTION ( 'NONE',  ( 1.000000000000000000, 0.000000000000000000, 0.000000000000000000 ) ) ;
#28029=EDGE_LOOP ( 'NONE', ( #16191, #30210, #31542, #16718 ) ) ;
#28037=ORIENTED_EDGE ( 'NONE', *, *, #2492, .F. ) ;
#28082=ORIENTED_EDGE ( 'NONE', *, *, #14738, .T. ) ;
#28088=VECTOR ( 'NONE', #33705, 1000.000000000000000 ) ;
#28099=EDGE_LOOP ( 'NONE', ( #21108, #29993, #27241, #19729 ) ) ;
#28179=ORIENTED_EDGE ( 'NONE', *, *, #15535, .F. ) ;
#28194=CARTESIAN_POINT ( 'NONE',  ( -39.49999999999999289, -1.387778780781445676E-14, 106.0000000000000000 ) ) ;
#28258=ORIENTED_EDGE ( 'NONE', *, *, #11092, .F. ) ;
#28323=UNCERTAINTY_MEASURE_WITH_UNIT (LENGTH_MEASURE( 1.000000000000000082E-05 ), #3166, 'distance_accuracy_value', 'NONE');
#28337=DIRECTION ( 'NONE',  ( 1.000000000000000000, 0.000000000000000000, 0.000000000000000000 ) ) ;
#28346=FILL_AREA_STYLE_COLOUR ( '', #31669 ) ;
#28348=VERTEX_POINT ( 'NONE', #5192 ) ;
#28383=VECTOR ( 'NONE', #25317, 1000.000000000000000 ) ;
#28436=EDGE_CURVE ( 'NONE', #31548, #33309, #28540, .T. ) ;
#28460=FACE_OUTER_BOUND ( 'NONE', #1416, .T. ) ;
#28494=CIRCLE ( 'NONE', #5501, 9.999999999999994671 ) ;
#28540=CIRCLE ( 'NONE', #33698, 9.999999999999994671 ) ;
#28550=AXIS2_PLACEMENT_3D ( 'NONE', #10681, #10865, #32110 ) ;
#28566=AXIS2_PLACEMENT_3D ( 'NONE', #19203, #30203, #24976 ) ;
#28625=EDGE_CURVE ( 'NONE', #1924, #26408, #22080, .T. ) ;
#28724=AXIS2_PLACEMENT_3D ( 'NONE', #21750, #18880, #34745 ) ;
#28874=DIRECTION ( 'NONE',  ( 1.000000000000000000, 0.000000000000000000, 0.000000000000000000 ) ) ;
#28876=CYLINDRICAL_SURFACE ( 'NONE', #32994, 4.000000000000003553 ) ;
#28974=ORIENTED_EDGE ( 'NONE', *, *, #29058, .F. ) ;
#28993=CYLINDRICAL_SURFACE ( 'NONE', #19218, 2.999999999999988898 ) ;
#28999=DIRECTION ( 'NONE',  ( 0.000000000000000000, 0.000000000000000000, -1.000000000000000000 ) ) ;
#29042=ORIENTED_EDGE ( 'NONE', *, *, #16342, .F. ) ;
#29058=EDGE_CURVE ( 'NONE', #11436, #28348, #995, .T. ) ;
#29133=DIRECTION ( 'NONE',  ( 0.000000000000000000, 0.5000000000000008882, -0.8660254037844382635 ) ) ;
#29169=DIRECTION ( 'NONE',  ( 1.000000000000000000, 0.000000000000000000, 0.000000000000000000 ) ) ;
#29196=ORIENTED_EDGE ( 'NONE', *, *, #5587, .F. ) ;
#29199=AXIS2_PLACEMENT_3D ( 'NONE', #16581, #5620, #25229 ) ;
#29202=DIRECTION ( 'NONE',  ( 1.000000000000000000, 0.000000000000000000, 0.000000000000000000 ) ) ;
#29235=VERTEX_POINT ( 'NONE', #27983 ) ;
#29243=CARTESIAN_POINT ( 'NONE',  ( -34.49999999999998579, -1.387778780781445676E-14, 110.0000000000000000 ) ) ;
#29276=CARTESIAN_POINT ( 'NONE',  ( -39.49999999999999289, -14.67619866229204284, 93.25874355921412473 ) ) ;
#29280=DIRECTION ( 'NONE',  ( 0.000000000000000000, 0.000000000000000000, -1.000000000000000000 ) ) ;
#29416=DIRECTION ( 'NONE',  ( 0.000000000000000000, 0.000000000000000000, -1.000000000000000000 ) ) ;
#29455=LINE ( 'NONE', #32149, #27343 ) ;
#29504=DIRECTION ( 'NONE',  ( -0.000000000000000000, 2.543449303551180694E-16, -1.000000000000000000 ) ) ;
#29548=ADVANCED_FACE ( 'NONE', ( #19599 ), #17078, .T. ) ;
#29580=CARTESIAN_POINT ( 'NONE',  ( -34.49999999999998579, -1.387778780781445676E-14, 110.0000000000000000 ) ) ;
#29623=CARTESIAN_POINT ( 'NONE',  ( -39.49999999999999289, -13.10640646055107084, 90.70096189432331357 ) ) ;
#29850=LINE ( 'NONE', #32717, #33065 ) ;
#29980=DIRECTION ( 'NONE',  ( 0.000000000000000000, 0.000000000000000000, -1.000000000000000000 ) ) ;
#29993=ORIENTED_EDGE ( 'NONE', *, *, #827, .T. ) ;
#30007=ADVANCED_FACE ( 'NONE', ( #22441 ), #309, .T. ) ;
#30038=FILL_AREA_STYLE ('',( #10589 ) ) ;
#30040=ORIENTED_EDGE ( 'NONE', *, *, #28436, .F. ) ;
#30188=PRODUCT_DEFINITION ( 'UNKNOWN', '', #24728, #22016 ) ;
#30202=DIRECTION ( 'NONE',  ( 1.000000000000000000, 0.000000000000000000, 0.000000000000000000 ) ) ;
#30203=DIRECTION ( 'NONE',  ( 1.000000000000000000, 0.000000000000000000, 0.000000000000000000 ) ) ;
#30210=ORIENTED_EDGE ( 'NONE', *, *, #27073, .T. ) ;
#30287=ORIENTED_EDGE ( 'NONE', *, *, #35203, .T. ) ;
#30311=ORIENTED_EDGE ( 'NONE', *, *, #27164, .T. ) ;
#30319=VECTOR ( 'NONE', #32902, 1000.000000000000000 ) ;
#30377=CARTESIAN_POINT ( 'NONE',  ( -37.49999999999999289, -11.52052244843579309, 112.1848168619253840 ) ) ;
#30481=DIRECTION ( 'NONE',  ( 0.000000000000000000, 0.000000000000000000, -1.000000000000000000 ) ) ;
#30550=LINE ( 'NONE', #24444, #6050 ) ;
#30738=PLANE ( 'NONE',  #27144 ) ;
#30749=DIRECTION ( 'NONE',  ( 0.000000000000000000, -3.469446951953611033E-15, -1.000000000000000000 ) ) ;
#30782=DIRECTION ( 'NONE',  ( 1.000000000000000000, 0.000000000000000000, 0.000000000000000000 ) ) ;
#30894=VECTOR ( 'NONE', #21717, 1000.000000000000000 ) ;
#30921=ORIENTED_EDGE ( 'NONE', *, *, #15535, .T. ) ;
#30946=ORIENTED_EDGE ( 'NONE', *, *, #18754, .F. ) ;
#30951=VECTOR ( 'NONE', #9663, 1000.000000000000000 ) ;
#30962=VERTEX_POINT ( 'NONE', #5427 ) ;
#30987=CARTESIAN_POINT ( 'NONE',  ( -39.49999999999999289, -3.784235812937200460, 96.08311962715481513 ) ) ;
#31088=VERTEX_POINT ( 'NONE', #16734 ) ;
#31093=ADVANCED_FACE ( 'NONE', ( #22662 ), #19770, .T. ) ;
#31115=CARTESIAN_POINT ( 'NONE',  ( -39.49999999999999289, -9.059673409587547965, 113.4689433211305811 ) ) ;
#31166=LINE ( 'NONE', #30987, #21632 ) ;
#31171=ORIENTED_EDGE ( 'NONE', *, *, #7245, .T. ) ;
#31195=UNCERTAINTY_MEASURE_WITH_UNIT (LENGTH_MEASURE( 1.000000000000000082E-05 ), #14468, 'distance_accuracy_value', 'NONE');
#31251=FACE_OUTER_BOUND ( 'NONE', #14085, .T. ) ;
#31310=AXIS2_PLACEMENT_3D ( 'NONE', #160, #25547, #24836 ) ;
#31535=ADVANCED_FACE ( 'NONE', ( #24989 ), #30738, .T. ) ;
#31539=LINE ( 'NONE', #4358, #20512 ) ;
#31542=ORIENTED_EDGE ( 'NONE', *, *, #25698, .F. ) ;
#31548=VERTEX_POINT ( 'NONE', #27864 ) ;
#31609=DIRECTION ( 'NONE',  ( 0.000000000000000000, 0.000000000000000000, -1.000000000000000000 ) ) ;
#31628=LINE ( 'NONE', #4113, #27553 ) ;
#31669=COLOUR_RGB ( '', 0.09019608, 0.27058824, 0.51372549) ;
#31718=ORIENTED_EDGE ( 'NONE', *, *, #32711, .F. ) ;
#31849=CARTESIAN_POINT ( 'NONE',  ( -39.49999999999999289, -14.17619866229204106, 94.12476896299857287 ) ) ;
#32095=VECTOR ( 'NONE', #7533, 1000.000000000000000 ) ;
#32105=DIRECTION ( 'NONE',  ( 0.000000000000000000, 0.000000000000000000, -1.000000000000000000 ) ) ;
#32110=DIRECTION ( 'NONE',  ( 0.000000000000000000, 0.000000000000000000, -1.000000000000000000 ) ) ;
#32149=CARTESIAN_POINT ( 'NONE',  ( -34.49999999999998579, -11.24969279549607748, 111.5585998451919778 ) ) ;
#32193=CARTESIAN_POINT ( 'NONE',  ( -34.49999999999998579, -12.31102132296306451, 91.73752798680880005 ) ) ;
#32244=VERTEX_POINT ( 'NONE', #24038 ) ;
#32283=LINE ( 'NONE', #7433, #6355 ) ;
#32289=EDGE_LOOP ( 'NONE', ( #21259, #2471, #24667, #6911, #11677, #5687, #34074 ) ) ;
#32472=LINE ( 'NONE', #5134, #11518 ) ;
#32539=PRESENTATION_STYLE_ASSIGNMENT (( #13470 ) ) ;
#32621=AXIS2_PLACEMENT_3D ( 'NONE', #33952, #11794, #17366 ) ;
#32711=EDGE_CURVE ( 'NONE', #13216, #26461, #6880, .T. ) ;
#32717=CARTESIAN_POINT ( 'NONE',  ( -39.49999999999999289, -11.24969279549607748, 111.5585998451919778 ) ) ;
#32719=CARTESIAN_POINT ( 'NONE',  ( -39.49999999999999289, -5.633167542791597704, 121.0048025873810218 ) ) ;
#32824=ORIENTED_EDGE ( 'NONE', *, *, #24701, .F. ) ;
#32852=DIRECTION ( 'NONE',  ( 0.000000000000000000, -0.9659258262890686453, 0.2588190451025194072 ) ) ;
#32863=ORIENTED_EDGE ( 'NONE', *, *, #20822, .T. ) ;
#32902=DIRECTION ( 'NONE',  ( 1.000000000000000000, 0.000000000000000000, 0.000000000000000000 ) ) ;
#32905=AXIS2_PLACEMENT_3D ( 'NONE', #1494, #23088, #20565 ) ;
#32994=AXIS2_PLACEMENT_3D ( 'NONE', #25651, #4229, #983 ) ;
#33029=PLANE ( 'NONE',  #1900 ) ;
#33049=EDGE_CURVE ( 'NONE', #34547, #14078, #17216, .T. ) ;
#33065=VECTOR ( 'NONE', #5006, 1000.000000000000000 ) ;
#33069=ADVANCED_FACE ( 'NONE', ( #8595 ), #16525, .T. ) ;
#33076=DIRECTION ( 'NONE',  ( 0.000000000000000000, 0.8660254037844379305, 0.5000000000000011102 ) ) ;
#33096=AXIS2_PLACEMENT_3D ( 'NONE', #13078, #23691, #4626 ) ;
#33101=CARTESIAN_POINT ( 'NONE',  ( -34.49999999999998579, -14.17619866229204106, 94.12476896299857287 ) ) ;
#33157=CARTESIAN_POINT ( 'NONE',  ( -39.49999999999999289, -14.67619866229204284, 94.12476896299857287 ) ) ;
#33188=DIRECTION ( 'NONE',  ( 1.000000000000000000, 0.000000000000000000, 0.000000000000000000 ) ) ;
#33219=CARTESIAN_POINT ( 'NONE',  ( -34.49999999999998579, -14.67619866229204284, 94.12476896299857287 ) ) ;
#33260=EDGE_LOOP ( 'NONE', ( #24991, #27476, #15088, #32824 ) ) ;
#33277=DIRECTION ( 'NONE',  ( 0.000000000000000000, 0.000000000000000000, -1.000000000000000000 ) ) ;
#33309=VERTEX_POINT ( 'NONE', #19853 ) ;
#33373=PLANE ( 'NONE',  #439 ) ;
#33431=DIRECTION ( 'NONE',  ( 0.000000000000000000, 0.8660254037844380415, 0.5000000000000012212 ) ) ;
#33441=DIRECTION ( 'NONE',  ( 1.000000000000000000, 0.000000000000000000, 0.000000000000000000 ) ) ;
#33492=DIRECTION ( 'NONE',  ( 1.000000000000000000, 0.000000000000000000, 0.000000000000000000 ) ) ;
#33557=CARTESIAN_POINT ( 'NONE',  ( -34.49999999999998579, -4.633167542791596816, 143.9590043477703887 ) ) ;
#33651=CARTESIAN_POINT ( 'NONE',  ( -39.49999999999999289, -14.17619866229204106, 94.12476896299857287 ) ) ;
#33661=AXIS2_PLACEMENT_3D ( 'NONE', #11759, #14628, #26163 ) ;
#33698=AXIS2_PLACEMENT_3D ( 'NONE', #15596, #21367, #34906 ) ;
#33705=DIRECTION ( 'NONE',  ( 1.000000000000000000, 0.000000000000000000, 0.000000000000000000 ) ) ;
#33724=FACE_BOUND ( 'NONE', #18987, .T. ) ;
#33769=CARTESIAN_POINT ( 'NONE',  ( -39.49999999999999289, 7.019851009788996343, 105.5074730863398003 ) ) ;
#33791=VERTEX_POINT ( 'NONE', #34915 ) ;
#33883=LINE ( 'NONE', #9212, #25161 ) ;
#33908=CYLINDRICAL_SURFACE ( 'NONE', #19120, 4.000000000000003553 ) ;
#33931=MANIFOLD_SOLID_BREP ( 'Fillet3', #6044 ) ;
#33945=EDGE_CURVE ( 'NONE', #12138, #17844, #2678, .T. ) ;
#33952=CARTESIAN_POINT ( 'NONE',  ( -39.49999999999999289, -12.31102132296306451, 91.73752798680880005 ) ) ;
#33958=SHAPE_REPRESENTATION ( 'Heavy-Duty Locking Pawl', ( #21307 ), #6954 ) ;
#33984=PRODUCT_CONTEXT ( 'NONE', #25960, 'mechanical' ) ;
#34074=ORIENTED_EDGE ( 'NONE', *, *, #19082, .F. ) ;
#34077=DIRECTION ( 'NONE',  ( 0.000000000000000000, -0.4387576694191720472, 0.8986054237126862576 ) ) ;
#34190=ORIENTED_EDGE ( 'NONE', *, *, #27495, .F. ) ;
#34281=FACE_OUTER_BOUND ( 'NONE', #28099, .T. ) ;
#34316=CARTESIAN_POINT ( 'NONE',  ( -37.49999999999999289, -11.52052244843579309, 115.1848168619253698 ) ) ;
#34424=VERTEX_POINT ( 'NONE', #5159 ) ;
#34498=DIRECTION ( 'NONE',  ( 0.000000000000000000, 0.8660254037844379305, 0.5000000000000011102 ) ) ;
#34535=DIRECTION ( 'NONE',  ( 0.000000000000000000, 0.8660254037844381525, 0.5000000000000007772 ) ) ;
#34547=VERTEX_POINT ( 'NONE', #33219 ) ;
#34567=CARTESIAN_POINT ( 'NONE',  ( -37.49999999999999289, -11.52052244843579309, 115.1848168619253698 ) ) ;
#34667=VECTOR ( 'NONE', #18998, 1000.000000000000227 ) ;
#34732=AXIS2_PLACEMENT_3D ( 'NONE', #2973, #24920, #8696 ) ;
#34745=DIRECTION ( 'NONE',  ( 0.000000000000000000, 0.000000000000000000, -1.000000000000000000 ) ) ;
#34763=EDGE_CURVE ( 'NONE', #13129, #32244, #19880, .T. ) ;
#34839=EDGE_CURVE ( 'NONE', #17814, #4619, #9585, .T. ) ;
#34853=EDGE_CURVE ( 'NONE', #16992, #31088, #20480, .T. ) ;
#34892=AXIS2_PLACEMENT_3D ( 'NONE', #20577, #28874, #15165 ) ;
#34906=DIRECTION ( 'NONE',  ( 0.000000000000000000, 0.000000000000000000, 1.000000000000000000 ) ) ;
#34915=CARTESIAN_POINT ( 'NONE',  ( -34.49999999999998579, 9.432411113711806294, 117.4309090467819772 ) ) ;
#34951=ORIENTED_EDGE ( 'NONE', *, *, #15018, .F. ) ;
#34991=DIRECTION ( 'NONE',  ( 0.000000000000000000, 0.000000000000000000, -1.000000000000000000 ) ) ;
#35008=ADVANCED_FACE ( 'NONE', ( #11559 ), #16600, .T. ) ;
#35139=AXIS2_PLACEMENT_3D ( 'NONE', #15630, #9402, #34077 ) ;
#35203=EDGE_CURVE ( 'NONE', #19887, #34547, #31539, .T. ) ;
#35312=ORIENTED_EDGE ( 'NONE', *, *, #4036, .F. ) ;
#35436=( NAMED_UNIT ( * ) PLANE_ANGLE_UNIT ( ) SI_UNIT ( $, .RADIAN. ) );
#35525=ORIENTED_EDGE ( 'NONE', *, *, #5734, .F. ) ;
#35596=DIRECTION ( 'NONE',  ( 0.000000000000000000, 0.7535859266250380939, 0.6573494133204066392 ) ) ;
#35606=DIRECTION ( 'NONE',  ( 0.000000000000000000, 0.000000000000000000, -1.000000000000000000 ) ) ;
ENDSEC;
END-ISO-10303-21;
